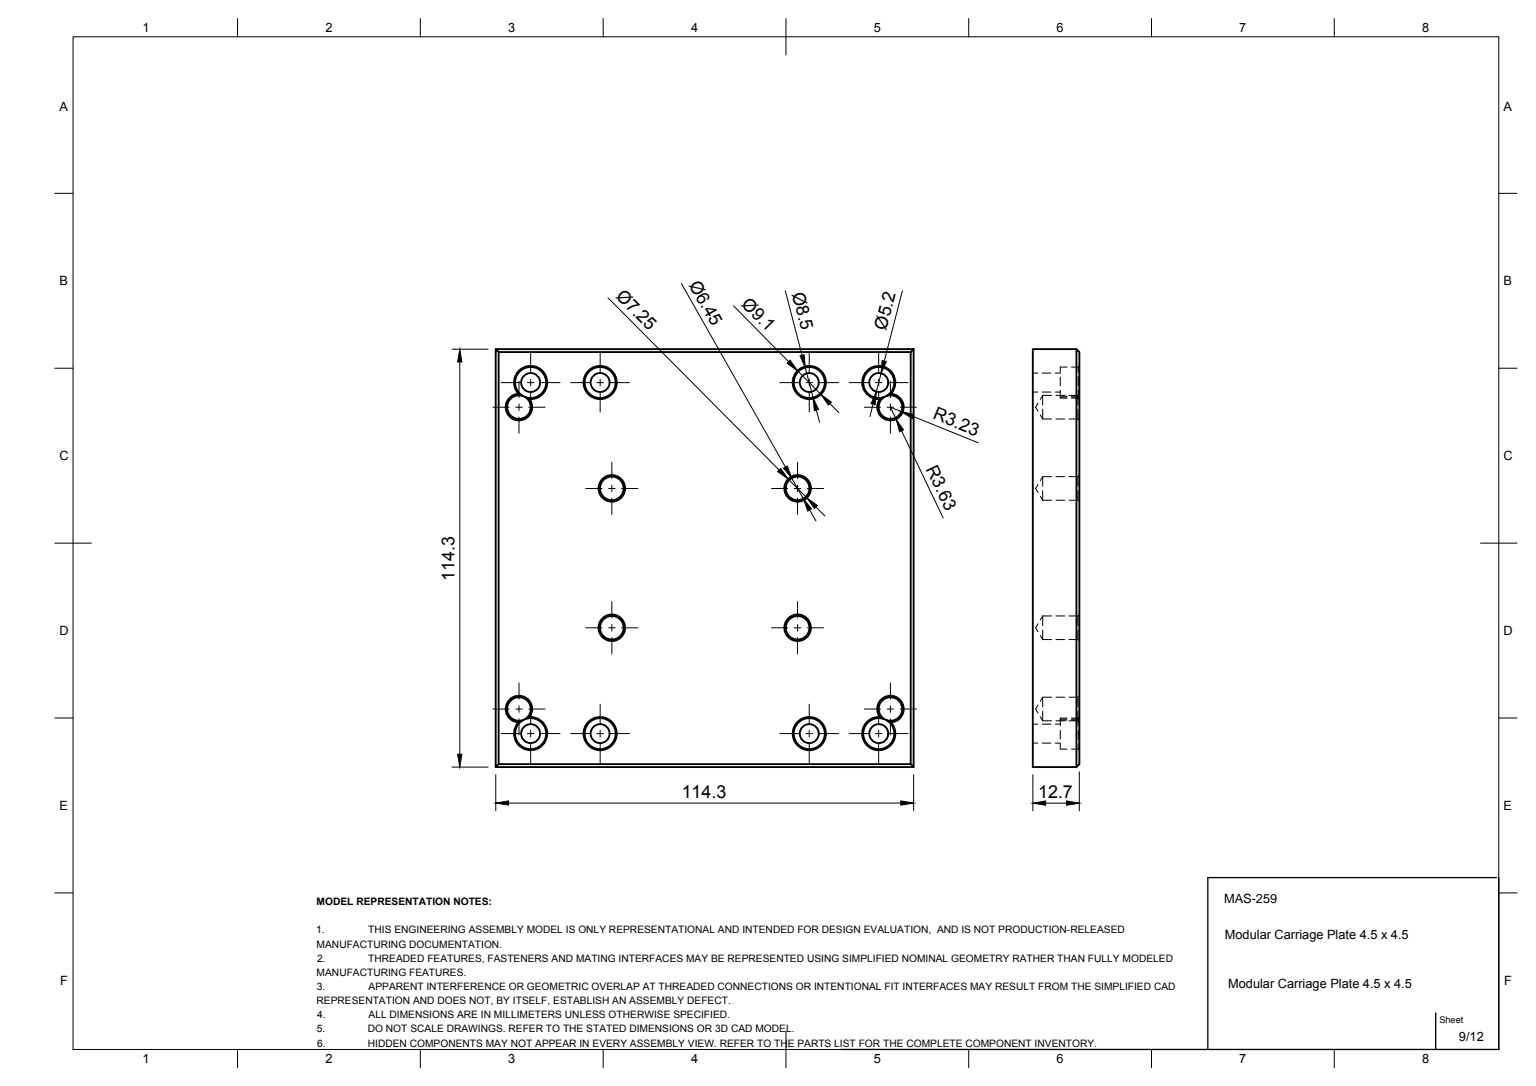
ISO-10303-21;
HEADER;
/* Generated by software containing ST-Developer
 * from STEP Tools, Inc. (www.steptools.com) 
 */

FILE_DESCRIPTION(
/* description */ (''),
/* implementation_level */ '2;1');

FILE_NAME(
/* name */ 'Modular Carriage Plate 4.5 x 4.5.step',
/* time_stamp */ '2026-10-15T13:30:17-07:00',
/* author */ (''),
/* organization */ (''),
/* preprocessor_version */ 'ST-DEVELOPER v20.2',
/* originating_system */ 'Autodesk Translation Framework v15.15.0.0',
/* authorisation */ '');

FILE_SCHEMA (('AUTOMOTIVE_DESIGN { 1 0 10303 214 3 1 1 }'));
ENDSEC;

DATA;
#10=MECHANICAL_DESIGN_GEOMETRIC_PRESENTATION_REPRESENTATION('',(#1034),#71795);
#1014=SHAPE_REPRESENTATION_RELATIONSHIP('SRR','None',#72018,#1024);
#1024=ADVANCED_BREP_SHAPE_REPRESENTATION('',(#1044),#71786);
#1034=STYLED_ITEM('',(#72077),#1044);
#1044=MANIFOLD_SOLID_BREP('Body1',#13636);
#1057=CONICAL_SURFACE('',#13855,4.40000000000001,0.785398163397447);
#1058=CONICAL_SURFACE('',#13874,4.4,0.785398163397434);
#1059=CONICAL_SURFACE('',#13878,4.4,0.78539816339744);
#1060=CONICAL_SURFACE('',#13880,4.4,0.785398163397448);
#1061=CONICAL_SURFACE('',#13884,4.4,0.78539816339744);
#1062=CONICAL_SURFACE('',#13886,4.4,0.785398163397448);
#1063=CONICAL_SURFACE('',#13890,4.4,0.785398163397434);
#1064=CONICAL_SURFACE('',#13894,4.40000000000001,0.785398163397447);
#1065=CONICAL_SURFACE('',#13924,3.42499999999999,0.785398163397437);
#1066=CONICAL_SURFACE('',#13927,3.425,0.785398163397448);
#1067=CONICAL_SURFACE('',#13930,3.425,0.785398163397448);
#1068=CONICAL_SURFACE('',#13933,3.42499999999999,0.785398163397437);
#1069=CONICAL_SURFACE('',#13952,3.42499999999999,0.785398163397437);
#1070=CONICAL_SURFACE('',#13956,3.425,0.785398163397448);
#1071=CONICAL_SURFACE('',#13968,3.425,0.785398163397448);
#1072=CONICAL_SURFACE('',#13972,3.42499999999999,0.785398163397437);
#1073=CONICAL_SURFACE('',#13976,3.225,1.02974425867665);
#1074=CONICAL_SURFACE('',#13977,3.225,1.02974425867665);
#1075=CONICAL_SURFACE('',#13978,3.225,1.02974425867665);
#1076=CONICAL_SURFACE('',#13979,3.225,1.02974425867665);
#1077=CONICAL_SURFACE('',#13980,3.22499999999998,1.02974425867665);
#1078=CONICAL_SURFACE('',#13981,3.22499999999998,1.02974425867665);
#1079=CONICAL_SURFACE('',#13982,3.225,1.02974425867665);
#1080=CONICAL_SURFACE('',#13983,3.225,1.02974425867665);
#1115=B_SPLINE_CURVE_WITH_KNOTS('',3,(#19006,#19007,#19008,#19009,#19010,
#19011),.UNSPECIFIED.,.F.,.F.,(4,2,4),(2.00778188532846,2.05631559190232,
2.12443391712942),.UNSPECIFIED.);
#1116=B_SPLINE_CURVE_WITH_KNOTS('',3,(#19015,#19016,#19017,#19018,#19019,
#19020),.UNSPECIFIED.,.F.,.F.,(4,2,4),(1.74660138399546,1.81470102727558,
1.86325481657749),.UNSPECIFIED.);
#1117=B_SPLINE_CURVE_WITH_KNOTS('',3,(#19070,#19071,#19072,#19073,#19074,
#19075),.UNSPECIFIED.,.F.,.F.,(4,2,4),(2.00778188532849,2.05631559190233,
2.1244339171294),.UNSPECIFIED.);
#1118=B_SPLINE_CURVE_WITH_KNOTS('',3,(#19077,#19078,#19079,#19080,#19081,
#19082),.UNSPECIFIED.,.F.,.F.,(4,2,4),(1.74660138399545,1.81470102727557,
1.86325481657748),.UNSPECIFIED.);
#1119=B_SPLINE_CURVE_WITH_KNOTS('',3,(#19094,#19095,#19096,#19097,#19098,
#19099),.UNSPECIFIED.,.F.,.F.,(4,2,4),(2.00778188532849,2.05631559190233,
2.12443391712941),.UNSPECIFIED.);
#1120=B_SPLINE_CURVE_WITH_KNOTS('',3,(#19101,#19102,#19103,#19104,#19105,
#19106),.UNSPECIFIED.,.F.,.F.,(4,2,4),(1.74660138399546,1.81470102727557,
1.86325481657748),.UNSPECIFIED.);
#1121=B_SPLINE_CURVE_WITH_KNOTS('',3,(#19126,#19127,#19128,#19129,#19130,
#19131),.UNSPECIFIED.,.F.,.F.,(4,2,4),(2.00778188532849,2.05631559190232,
2.1244339171294),.UNSPECIFIED.);
#1122=B_SPLINE_CURVE_WITH_KNOTS('',3,(#19133,#19134,#19135,#19136,#19137,
#19138),.UNSPECIFIED.,.F.,.F.,(4,2,4),(1.74660138399543,1.81470102727559,
1.86325481657752),.UNSPECIFIED.);
#1123=B_SPLINE_CURVE_WITH_KNOTS('',3,(#19142,#19143,#19144,#19145),
 .UNSPECIFIED.,.F.,.F.,(4,4),(-0.456883774528942,-0.419587727931792),
 .UNSPECIFIED.);
#1124=B_SPLINE_CURVE_WITH_KNOTS('',3,(#19152,#19153,#19154,#19155),
 .UNSPECIFIED.,.F.,.F.,(4,4),(-0.557381628443529,-0.520085581846348),
 .UNSPECIFIED.);
#1125=B_SPLINE_CURVE_WITH_KNOTS('',3,(#19168,#19169,#19170,#19171),
 .UNSPECIFIED.,.F.,.F.,(4,4),(-0.456883774528974,-0.419587727931764),
 .UNSPECIFIED.);
#1126=B_SPLINE_CURVE_WITH_KNOTS('',3,(#19178,#19179,#19180,#19181),
 .UNSPECIFIED.,.F.,.F.,(4,4),(-0.557381628443525,-0.520085581846325),
 .UNSPECIFIED.);
#1127=B_SPLINE_CURVE_WITH_KNOTS('',3,(#19191,#19192,#19193,#19194),
 .UNSPECIFIED.,.F.,.F.,(4,4),(-0.456883774528968,-0.419587727931769),
 .UNSPECIFIED.);
#1128=B_SPLINE_CURVE_WITH_KNOTS('',3,(#19201,#19202,#19203,#19204),
 .UNSPECIFIED.,.F.,.F.,(4,4),(-0.557381628443528,-0.52008558184632),
 .UNSPECIFIED.);
#1129=B_SPLINE_CURVE_WITH_KNOTS('',3,(#19214,#19215,#19216,#19217),
 .UNSPECIFIED.,.F.,.F.,(4,4),(-0.456883774528947,-0.419587727931763),
 .UNSPECIFIED.);
#1130=B_SPLINE_CURVE_WITH_KNOTS('',3,(#19224,#19225,#19226,#19227),
 .UNSPECIFIED.,.F.,.F.,(4,4),(-0.557381628443516,-0.520085581846359),
 .UNSPECIFIED.);
#1514=FACE_BOUND('',#2761,.T.);
#1515=FACE_BOUND('',#2762,.T.);
#1516=FACE_BOUND('',#2763,.T.);
#1517=FACE_BOUND('',#2764,.T.);
#1518=FACE_BOUND('',#2765,.T.);
#1519=FACE_BOUND('',#2766,.T.);
#1520=FACE_BOUND('',#2767,.T.);
#1521=FACE_BOUND('',#2768,.T.);
#1522=FACE_BOUND('',#2769,.T.);
#1523=FACE_BOUND('',#2770,.T.);
#1524=FACE_BOUND('',#2771,.T.);
#1525=FACE_BOUND('',#2772,.T.);
#1526=FACE_BOUND('',#2786,.T.);
#1527=FACE_BOUND('',#2788,.T.);
#1528=FACE_BOUND('',#2790,.T.);
#1529=FACE_BOUND('',#2793,.T.);
#1530=FACE_BOUND('',#2795,.T.);
#1531=FACE_BOUND('',#2798,.T.);
#1532=FACE_BOUND('',#2800,.T.);
#1533=FACE_BOUND('',#2803,.T.);
#1534=FACE_BOUND('',#2845,.T.);
#1535=FACE_BOUND('',#2846,.T.);
#1536=FACE_BOUND('',#2847,.T.);
#1537=FACE_BOUND('',#2848,.T.);
#1538=FACE_BOUND('',#2849,.T.);
#1539=FACE_BOUND('',#2850,.T.);
#1540=FACE_BOUND('',#2851,.T.);
#1541=FACE_BOUND('',#2852,.T.);
#1593=PLANE('',#13858);
#1594=PLANE('',#13898);
#1595=PLANE('',#13901);
#1596=PLANE('',#13903);
#1597=PLANE('',#13907);
#1598=PLANE('',#13910);
#1599=PLANE('',#13914);
#1600=PLANE('',#13917);
#1601=PLANE('',#13921);
#1602=PLANE('',#13984);
#1603=PLANE('',#13985);
#1604=PLANE('',#13986);
#1605=PLANE('',#13987);
#1606=PLANE('',#13988);
#1607=PLANE('',#13989);
#1608=PLANE('',#13990);
#1609=PLANE('',#13991);
#1610=PLANE('',#13992);
#2081=FACE_OUTER_BOUND('',#2759,.T.);
#2082=FACE_OUTER_BOUND('',#2760,.T.);
#2083=FACE_OUTER_BOUND('',#2773,.T.);
#2084=FACE_OUTER_BOUND('',#2774,.T.);
#2085=FACE_OUTER_BOUND('',#2775,.T.);
#2086=FACE_OUTER_BOUND('',#2776,.T.);
#2087=FACE_OUTER_BOUND('',#2777,.T.);
#2088=FACE_OUTER_BOUND('',#2778,.T.);
#2089=FACE_OUTER_BOUND('',#2779,.T.);
#2090=FACE_OUTER_BOUND('',#2780,.T.);
#2091=FACE_OUTER_BOUND('',#2781,.T.);
#2092=FACE_OUTER_BOUND('',#2782,.T.);
#2093=FACE_OUTER_BOUND('',#2783,.T.);
#2094=FACE_OUTER_BOUND('',#2784,.T.);
#2095=FACE_OUTER_BOUND('',#2785,.T.);
#2096=FACE_OUTER_BOUND('',#2787,.T.);
#2097=FACE_OUTER_BOUND('',#2789,.T.);
#2098=FACE_OUTER_BOUND('',#2791,.T.);
#2099=FACE_OUTER_BOUND('',#2792,.T.);
#2100=FACE_OUTER_BOUND('',#2794,.T.);
#2101=FACE_OUTER_BOUND('',#2796,.T.);
#2102=FACE_OUTER_BOUND('',#2797,.T.);
#2103=FACE_OUTER_BOUND('',#2799,.T.);
#2104=FACE_OUTER_BOUND('',#2801,.T.);
#2105=FACE_OUTER_BOUND('',#2802,.T.);
#2106=FACE_OUTER_BOUND('',#2804,.T.);
#2107=FACE_OUTER_BOUND('',#2805,.T.);
#2108=FACE_OUTER_BOUND('',#2806,.T.);
#2109=FACE_OUTER_BOUND('',#2807,.T.);
#2110=FACE_OUTER_BOUND('',#2808,.T.);
#2111=FACE_OUTER_BOUND('',#2809,.T.);
#2112=FACE_OUTER_BOUND('',#2810,.T.);
#2113=FACE_OUTER_BOUND('',#2811,.T.);
#2114=FACE_OUTER_BOUND('',#2812,.T.);
#2115=FACE_OUTER_BOUND('',#2813,.T.);
#2116=FACE_OUTER_BOUND('',#2814,.T.);
#2117=FACE_OUTER_BOUND('',#2815,.T.);
#2118=FACE_OUTER_BOUND('',#2816,.T.);
#2119=FACE_OUTER_BOUND('',#2817,.T.);
#2120=FACE_OUTER_BOUND('',#2818,.T.);
#2121=FACE_OUTER_BOUND('',#2819,.T.);
#2122=FACE_OUTER_BOUND('',#2820,.T.);
#2123=FACE_OUTER_BOUND('',#2821,.T.);
#2124=FACE_OUTER_BOUND('',#2822,.T.);
#2125=FACE_OUTER_BOUND('',#2823,.T.);
#2126=FACE_OUTER_BOUND('',#2824,.T.);
#2127=FACE_OUTER_BOUND('',#2825,.T.);
#2128=FACE_OUTER_BOUND('',#2826,.T.);
#2129=FACE_OUTER_BOUND('',#2827,.T.);
#2130=FACE_OUTER_BOUND('',#2828,.T.);
#2131=FACE_OUTER_BOUND('',#2829,.T.);
#2132=FACE_OUTER_BOUND('',#2830,.T.);
#2133=FACE_OUTER_BOUND('',#2831,.T.);
#2134=FACE_OUTER_BOUND('',#2832,.T.);
#2135=FACE_OUTER_BOUND('',#2833,.T.);
#2136=FACE_OUTER_BOUND('',#2834,.T.);
#2137=FACE_OUTER_BOUND('',#2835,.T.);
#2138=FACE_OUTER_BOUND('',#2836,.T.);
#2139=FACE_OUTER_BOUND('',#2837,.T.);
#2140=FACE_OUTER_BOUND('',#2838,.T.);
#2141=FACE_OUTER_BOUND('',#2839,.T.);
#2142=FACE_OUTER_BOUND('',#2840,.T.);
#2143=FACE_OUTER_BOUND('',#2841,.T.);
#2144=FACE_OUTER_BOUND('',#2842,.T.);
#2145=FACE_OUTER_BOUND('',#2843,.T.);
#2146=FACE_OUTER_BOUND('',#2844,.T.);
#2759=EDGE_LOOP('',(#9221,#9222,#9223,#9224));
#2760=EDGE_LOOP('',(#9225,#9226,#9227,#9228));
#2761=EDGE_LOOP('',(#9229));
#2762=EDGE_LOOP('',(#9230));
#2763=EDGE_LOOP('',(#9231));
#2764=EDGE_LOOP('',(#9232));
#2765=EDGE_LOOP('',(#9233,#9234));
#2766=EDGE_LOOP('',(#9235,#9236));
#2767=EDGE_LOOP('',(#9237));
#2768=EDGE_LOOP('',(#9238));
#2769=EDGE_LOOP('',(#9239,#9240));
#2770=EDGE_LOOP('',(#9241,#9242));
#2771=EDGE_LOOP('',(#9243));
#2772=EDGE_LOOP('',(#9244));
#2773=EDGE_LOOP('',(#9245,#9246,#9247,#9248));
#2774=EDGE_LOOP('',(#9249,#9250,#9251,#9252));
#2775=EDGE_LOOP('',(#9253,#9254,#9255,#9256));
#2776=EDGE_LOOP('',(#9257,#9258,#9259,#9260));
#2777=EDGE_LOOP('',(#9261,#9262,#9263,#9264));
#2778=EDGE_LOOP('',(#9265,#9266,#9267,#9268));
#2779=EDGE_LOOP('',(#9269,#9270,#9271,#9272));
#2780=EDGE_LOOP('',(#9273,#9274,#9275,#9276));
#2781=EDGE_LOOP('',(#9277,#9278,#9279,#9280));
#2782=EDGE_LOOP('',(#9281,#9282,#9283,#9284));
#2783=EDGE_LOOP('',(#9285,#9286,#9287,#9288));
#2784=EDGE_LOOP('',(#9289,#9290,#9291,#9292,#9293,#9294));
#2785=EDGE_LOOP('',(#9295,#9296));
#2786=EDGE_LOOP('',(#9297));
#2787=EDGE_LOOP('',(#9298));
#2788=EDGE_LOOP('',(#9299));
#2789=EDGE_LOOP('',(#9300));
#2790=EDGE_LOOP('',(#9301));
#2791=EDGE_LOOP('',(#9302,#9303,#9304,#9305,#9306,#9307));
#2792=EDGE_LOOP('',(#9308,#9309));
#2793=EDGE_LOOP('',(#9310));
#2794=EDGE_LOOP('',(#9311));
#2795=EDGE_LOOP('',(#9312));
#2796=EDGE_LOOP('',(#9313,#9314,#9315,#9316,#9317,#9318));
#2797=EDGE_LOOP('',(#9319,#9320));
#2798=EDGE_LOOP('',(#9321));
#2799=EDGE_LOOP('',(#9322));
#2800=EDGE_LOOP('',(#9323));
#2801=EDGE_LOOP('',(#9324,#9325,#9326,#9327,#9328,#9329));
#2802=EDGE_LOOP('',(#9330,#9331));
#2803=EDGE_LOOP('',(#9332));
#2804=EDGE_LOOP('',(#9333,#9334,#9335,#9336,#9337,#9338,#9339));
#2805=EDGE_LOOP('',(#9340,#9341,#9342,#9343,#9344,#9345,#9346));
#2806=EDGE_LOOP('',(#9347,#9348,#9349,#9350,#9351,#9352,#9353));
#2807=EDGE_LOOP('',(#9354,#9355,#9356,#9357,#9358,#9359,#9360));
#2808=EDGE_LOOP('',(#9361,#9362,#9363,#9364));
#2809=EDGE_LOOP('',(#9365,#9366,#9367,#9368));
#2810=EDGE_LOOP('',(#9369,#9370,#9371,#9372));
#2811=EDGE_LOOP('',(#9373,#9374,#9375,#9376));
#2812=EDGE_LOOP('',(#9377,#9378,#9379,#9380));
#2813=EDGE_LOOP('',(#9381,#9382,#9383,#9384));
#2814=EDGE_LOOP('',(#9385,#9386,#9387,#9388));
#2815=EDGE_LOOP('',(#9389,#9390,#9391,#9392));
#2816=EDGE_LOOP('',(#9393,#9394,#9395,#9396));
#2817=EDGE_LOOP('',(#9397,#9398,#9399,#9400));
#2818=EDGE_LOOP('',(#9401,#9402,#9403,#9404));
#2819=EDGE_LOOP('',(#9405,#9406,#9407,#9408));
#2820=EDGE_LOOP('',(#9409,#9410,#9411,#9412,#9413,#9414,#9415,#9416));
#2821=EDGE_LOOP('',(#9417,#9418,#9419,#9420,#9421,#9422,#9423,#9424));
#2822=EDGE_LOOP('',(#9425,#9426,#9427,#9428,#9429,#9430,#9431,#9432));
#2823=EDGE_LOOP('',(#9433,#9434,#9435,#9436,#9437,#9438,#9439,#9440));
#2824=EDGE_LOOP('',(#9441,#9442,#9443,#9444));
#2825=EDGE_LOOP('',(#9445,#9446,#9447,#9448));
#2826=EDGE_LOOP('',(#9449,#9450,#9451,#9452));
#2827=EDGE_LOOP('',(#9453,#9454,#9455,#9456));
#2828=EDGE_LOOP('',(#9457,#9458,#9459));
#2829=EDGE_LOOP('',(#9460,#9461,#9462));
#2830=EDGE_LOOP('',(#9463,#9464,#9465));
#2831=EDGE_LOOP('',(#9466,#9467,#9468));
#2832=EDGE_LOOP('',(#9469,#9470,#9471));
#2833=EDGE_LOOP('',(#9472,#9473,#9474));
#2834=EDGE_LOOP('',(#9475,#9476,#9477));
#2835=EDGE_LOOP('',(#9478,#9479,#9480));
#2836=EDGE_LOOP('',(#9481,#9482,#9483,#9484));
#2837=EDGE_LOOP('',(#9485,#9486,#9487,#9488));
#2838=EDGE_LOOP('',(#9489,#9490,#9491,#9492));
#2839=EDGE_LOOP('',(#9493,#9494,#9495,#9496));
#2840=EDGE_LOOP('',(#9497,#9498,#9499,#9500));
#2841=EDGE_LOOP('',(#9501,#9502,#9503,#9504));
#2842=EDGE_LOOP('',(#9505,#9506,#9507,#9508));
#2843=EDGE_LOOP('',(#9509,#9510,#9511,#9512));
#2844=EDGE_LOOP('',(#9513,#9514,#9515,#9516));
#2845=EDGE_LOOP('',(#9517));
#2846=EDGE_LOOP('',(#9518));
#2847=EDGE_LOOP('',(#9519));
#2848=EDGE_LOOP('',(#9520));
#2849=EDGE_LOOP('',(#9521));
#2850=EDGE_LOOP('',(#9522));
#2851=EDGE_LOOP('',(#9523));
#2852=EDGE_LOOP('',(#9524));
#3440=CIRCLE('',#13856,4.55000000000001);
#3441=CIRCLE('',#13857,4.25000000000001);
#3442=CIRCLE('',#13859,4.55);
#3443=CIRCLE('',#13860,4.55);
#3444=CIRCLE('',#13861,4.55);
#3445=CIRCLE('',#13862,3.625);
#3446=CIRCLE('',#13863,4.55000000000001);
#3447=CIRCLE('',#13864,3.62499999999999);
#3448=CIRCLE('',#13865,3.62499999999999);
#3449=CIRCLE('',#13866,3.62499999999999);
#3450=CIRCLE('',#13867,3.625);
#3451=CIRCLE('',#13868,4.55);
#3452=CIRCLE('',#13869,3.625);
#3453=CIRCLE('',#13870,4.55);
#3454=CIRCLE('',#13871,3.625);
#3455=CIRCLE('',#13872,3.62499999999999);
#3456=CIRCLE('',#13873,4.55);
#3457=CIRCLE('',#13875,4.25000000000001);
#3458=CIRCLE('',#13877,4.25000000000001);
#3459=CIRCLE('',#13879,4.25);
#3460=CIRCLE('',#13881,4.25);
#3461=CIRCLE('',#13883,4.25);
#3462=CIRCLE('',#13885,4.25);
#3463=CIRCLE('',#13887,4.25);
#3464=CIRCLE('',#13889,4.25);
#3465=CIRCLE('',#13891,4.25000000000001);
#3466=CIRCLE('',#13893,4.25000000000001);
#3467=CIRCLE('',#13895,4.25000000000001);
#3468=CIRCLE('',#13897,4.25000000000001);
#3469=CIRCLE('',#13899,3.225);
#3470=CIRCLE('',#13900,2.6);
#3471=CIRCLE('',#13902,2.6);
#3472=CIRCLE('',#13904,2.6);
#3473=CIRCLE('',#13906,4.25);
#3474=CIRCLE('',#13908,3.225);
#3475=CIRCLE('',#13909,2.6);
#3476=CIRCLE('',#13911,2.6);
#3477=CIRCLE('',#13913,4.25);
#3478=CIRCLE('',#13915,3.225);
#3479=CIRCLE('',#13916,2.6);
#3480=CIRCLE('',#13918,2.6);
#3481=CIRCLE('',#13920,4.25000000000001);
#3482=CIRCLE('',#13922,3.225);
#3483=CIRCLE('',#13923,2.6);
#3484=CIRCLE('',#13925,3.225);
#3485=CIRCLE('',#13926,3.225);
#3486=CIRCLE('',#13928,3.225);
#3487=CIRCLE('',#13929,3.225);
#3488=CIRCLE('',#13931,3.225);
#3489=CIRCLE('',#13932,3.225);
#3490=CIRCLE('',#13934,3.225);
#3491=CIRCLE('',#13935,3.225);
#3492=CIRCLE('',#13937,2.6);
#3493=CIRCLE('',#13939,2.6);
#3494=CIRCLE('',#13941,2.6);
#3495=CIRCLE('',#13943,2.6);
#3496=CIRCLE('',#13945,2.6);
#3497=CIRCLE('',#13947,2.6);
#3498=CIRCLE('',#13949,2.6);
#3499=CIRCLE('',#13951,2.6);
#3500=CIRCLE('',#13953,3.225);
#3501=CIRCLE('',#13955,3.225);
#3502=CIRCLE('',#13957,3.225);
#3503=CIRCLE('',#13959,3.225);
#3504=CIRCLE('',#13961,3.225);
#3505=CIRCLE('',#13963,3.225);
#3506=CIRCLE('',#13965,3.225);
#3507=CIRCLE('',#13967,3.225);
#3508=CIRCLE('',#13969,3.225);
#3509=CIRCLE('',#13971,3.225);
#3510=CIRCLE('',#13973,3.225);
#3511=CIRCLE('',#13975,3.225);
#3912=LINE('',#19025,#4823);
#3913=LINE('',#19027,#4824);
#3914=LINE('',#19029,#4825);
#3915=LINE('',#19030,#4826);
#3916=LINE('',#19063,#4827);
#3917=LINE('',#19066,#4828);
#3918=LINE('',#19087,#4829);
#3919=LINE('',#19090,#4830);
#3920=LINE('',#19111,#4831);
#3921=LINE('',#19114,#4832);
#3922=LINE('',#19119,#4833);
#3923=LINE('',#19122,#4834);
#3924=LINE('',#19147,#4835);
#3925=LINE('',#19151,#4836);
#3926=LINE('',#19173,#4837);
#3927=LINE('',#19177,#4838);
#3928=LINE('',#19196,#4839);
#3929=LINE('',#19200,#4840);
#3930=LINE('',#19219,#4841);
#3931=LINE('',#19223,#4842);
#3932=LINE('',#19250,#4843);
#3933=LINE('',#19254,#4844);
#3934=LINE('',#19258,#4845);
#3935=LINE('',#19262,#4846);
#3936=LINE('',#19266,#4847);
#3937=LINE('',#19270,#4848);
#3938=LINE('',#19274,#4849);
#3939=LINE('',#19278,#4850);
#3940=LINE('',#19283,#4851);
#3941=LINE('',#19286,#4852);
#3942=LINE('',#19291,#4853);
#3943=LINE('',#19294,#4854);
#3944=LINE('',#19298,#4855);
#3945=LINE('',#19302,#4856);
#3946=LINE('',#19306,#4857);
#3947=LINE('',#19310,#4858);
#3948=LINE('',#19315,#4859);
#3949=LINE('',#19318,#4860);
#3950=LINE('',#19323,#4861);
#3951=LINE('',#19326,#4862);
#3952=LINE('',#19330,#4863);
#3953=LINE('',#19333,#4864);
#3954=LINE('',#19336,#4865);
#3955=LINE('',#19339,#4866);
#3956=LINE('',#19342,#4867);
#3957=LINE('',#19345,#4868);
#3958=LINE('',#19348,#4869);
#3959=LINE('',#19351,#4870);
#3960=LINE('',#19354,#4871);
#3961=LINE('',#19356,#4872);
#3962=LINE('',#19357,#4873);
#3963=LINE('',#19360,#4874);
#3964=LINE('',#19361,#4875);
#3965=LINE('',#19364,#4876);
#3966=LINE('',#19365,#4877);
#3967=LINE('',#19367,#4878);
#3968=LINE('',#19370,#4879);
#3969=LINE('',#19372,#4880);
#3970=LINE('',#19373,#4881);
#3971=LINE('',#19376,#4882);
#3972=LINE('',#19377,#4883);
#3973=LINE('',#19380,#4884);
#3974=LINE('',#19381,#4885);
#3975=LINE('',#19383,#4886);
#4823=VECTOR('',#15323,10.);
#4824=VECTOR('',#15324,10.);
#4825=VECTOR('',#15325,10.);
#4826=VECTOR('',#15326,10.);
#4827=VECTOR('',#15361,4.4);
#4828=VECTOR('',#15364,4.25000000000001);
#4829=VECTOR('',#15375,4.4);
#4830=VECTOR('',#15378,4.25);
#4831=VECTOR('',#15389,4.4);
#4832=VECTOR('',#15392,4.25);
#4833=VECTOR('',#15399,4.4);
#4834=VECTOR('',#15402,4.25000000000001);
#4835=VECTOR('',#15411,10.);
#4836=VECTOR('',#15414,10.);
#4837=VECTOR('',#15431,10.);
#4838=VECTOR('',#15434,10.);
#4839=VECTOR('',#15447,10.);
#4840=VECTOR('',#15450,10.);
#4841=VECTOR('',#15463,10.);
#4842=VECTOR('',#15466,10.);
#4843=VECTOR('',#15499,2.6);
#4844=VECTOR('',#15504,2.6);
#4845=VECTOR('',#15509,2.6);
#4846=VECTOR('',#15514,2.6);
#4847=VECTOR('',#15519,2.6);
#4848=VECTOR('',#15524,2.6);
#4849=VECTOR('',#15529,2.6);
#4850=VECTOR('',#15534,2.6);
#4851=VECTOR('',#15541,3.42499999999999);
#4852=VECTOR('',#15544,3.225);
#4853=VECTOR('',#15551,3.425);
#4854=VECTOR('',#15554,3.225);
#4855=VECTOR('',#15559,3.225);
#4856=VECTOR('',#15564,3.225);
#4857=VECTOR('',#15569,3.225);
#4858=VECTOR('',#15574,3.225);
#4859=VECTOR('',#15581,3.425);
#4860=VECTOR('',#15584,3.225);
#4861=VECTOR('',#15591,3.42499999999999);
#4862=VECTOR('',#15594,3.225);
#4863=VECTOR('',#15599,3.225);
#4864=VECTOR('',#15602,3.225);
#4865=VECTOR('',#15605,3.225);
#4866=VECTOR('',#15608,3.225);
#4867=VECTOR('',#15611,3.22499999999998);
#4868=VECTOR('',#15614,3.22499999999998);
#4869=VECTOR('',#15617,3.225);
#4870=VECTOR('',#15620,3.225);
#4871=VECTOR('',#15623,10.);
#4872=VECTOR('',#15624,10.);
#4873=VECTOR('',#15625,10.);
#4874=VECTOR('',#15628,10.);
#4875=VECTOR('',#15629,10.);
#4876=VECTOR('',#15632,10.);
#4877=VECTOR('',#15633,10.);
#4878=VECTOR('',#15636,10.);
#4879=VECTOR('',#15639,10.);
#4880=VECTOR('',#15640,10.);
#4881=VECTOR('',#15641,10.);
#4882=VECTOR('',#15644,10.);
#4883=VECTOR('',#15645,10.);
#4884=VECTOR('',#15648,10.);
#4885=VECTOR('',#15649,10.);
#4886=VECTOR('',#15652,10.);
#5752=VERTEX_POINT('',#19004);
#5753=VERTEX_POINT('',#19005);
#5754=VERTEX_POINT('',#19012);
#5755=VERTEX_POINT('',#19014);
#5756=VERTEX_POINT('',#19023);
#5757=VERTEX_POINT('',#19024);
#5758=VERTEX_POINT('',#19026);
#5759=VERTEX_POINT('',#19028);
#5760=VERTEX_POINT('',#19031);
#5761=VERTEX_POINT('',#19033);
#5762=VERTEX_POINT('',#19035);
#5763=VERTEX_POINT('',#19037);
#5764=VERTEX_POINT('',#19039);
#5765=VERTEX_POINT('',#19040);
#5766=VERTEX_POINT('',#19044);
#5767=VERTEX_POINT('',#19046);
#5768=VERTEX_POINT('',#19048);
#5769=VERTEX_POINT('',#19049);
#5770=VERTEX_POINT('',#19052);
#5771=VERTEX_POINT('',#19053);
#5772=VERTEX_POINT('',#19056);
#5773=VERTEX_POINT('',#19058);
#5774=VERTEX_POINT('',#19061);
#5775=VERTEX_POINT('',#19065);
#5776=VERTEX_POINT('',#19069);
#5777=VERTEX_POINT('',#19076);
#5778=VERTEX_POINT('',#19085);
#5779=VERTEX_POINT('',#19089);
#5780=VERTEX_POINT('',#19093);
#5781=VERTEX_POINT('',#19100);
#5782=VERTEX_POINT('',#19109);
#5783=VERTEX_POINT('',#19113);
#5784=VERTEX_POINT('',#19117);
#5785=VERTEX_POINT('',#19121);
#5786=VERTEX_POINT('',#19125);
#5787=VERTEX_POINT('',#19132);
#5788=VERTEX_POINT('',#19141);
#5789=VERTEX_POINT('',#19146);
#5790=VERTEX_POINT('',#19148);
#5791=VERTEX_POINT('',#19150);
#5792=VERTEX_POINT('',#19158);
#5793=VERTEX_POINT('',#19161);
#5794=VERTEX_POINT('',#19164);
#5795=VERTEX_POINT('',#19167);
#5796=VERTEX_POINT('',#19172);
#5797=VERTEX_POINT('',#19174);
#5798=VERTEX_POINT('',#19176);
#5799=VERTEX_POINT('',#19184);
#5800=VERTEX_POINT('',#19187);
#5801=VERTEX_POINT('',#19190);
#5802=VERTEX_POINT('',#19195);
#5803=VERTEX_POINT('',#19197);
#5804=VERTEX_POINT('',#19199);
#5805=VERTEX_POINT('',#19207);
#5806=VERTEX_POINT('',#19210);
#5807=VERTEX_POINT('',#19213);
#5808=VERTEX_POINT('',#19218);
#5809=VERTEX_POINT('',#19220);
#5810=VERTEX_POINT('',#19222);
#5811=VERTEX_POINT('',#19230);
#5812=VERTEX_POINT('',#19233);
#5813=VERTEX_POINT('',#19237);
#5814=VERTEX_POINT('',#19241);
#5815=VERTEX_POINT('',#19245);
#5816=VERTEX_POINT('',#19249);
#5817=VERTEX_POINT('',#19253);
#5818=VERTEX_POINT('',#19257);
#5819=VERTEX_POINT('',#19261);
#5820=VERTEX_POINT('',#19265);
#5821=VERTEX_POINT('',#19269);
#5822=VERTEX_POINT('',#19273);
#5823=VERTEX_POINT('',#19277);
#5824=VERTEX_POINT('',#19281);
#5825=VERTEX_POINT('',#19285);
#5826=VERTEX_POINT('',#19289);
#5827=VERTEX_POINT('',#19293);
#5828=VERTEX_POINT('',#19297);
#5829=VERTEX_POINT('',#19301);
#5830=VERTEX_POINT('',#19305);
#5831=VERTEX_POINT('',#19309);
#5832=VERTEX_POINT('',#19313);
#5833=VERTEX_POINT('',#19317);
#5834=VERTEX_POINT('',#19321);
#5835=VERTEX_POINT('',#19325);
#5836=VERTEX_POINT('',#19329);
#5837=VERTEX_POINT('',#19332);
#5838=VERTEX_POINT('',#19335);
#5839=VERTEX_POINT('',#19338);
#5840=VERTEX_POINT('',#19341);
#5841=VERTEX_POINT('',#19344);
#5842=VERTEX_POINT('',#19347);
#5843=VERTEX_POINT('',#19350);
#5844=VERTEX_POINT('',#19353);
#5845=VERTEX_POINT('',#19355);
#5846=VERTEX_POINT('',#19359);
#5847=VERTEX_POINT('',#19363);
#5848=VERTEX_POINT('',#19369);
#5849=VERTEX_POINT('',#19371);
#5850=VERTEX_POINT('',#19375);
#5851=VERTEX_POINT('',#19379);
#7145=EDGE_CURVE('',#5752,#5753,#1115,.T.);
#7146=EDGE_CURVE('',#5753,#5754,#3440,.T.);
#7147=EDGE_CURVE('',#5754,#5755,#1116,.T.);
#7148=EDGE_CURVE('',#5755,#5752,#3441,.T.);
#7149=EDGE_CURVE('',#5756,#5757,#3912,.T.);
#7150=EDGE_CURVE('',#5758,#5756,#3913,.T.);
#7151=EDGE_CURVE('',#5759,#5758,#3914,.T.);
#7152=EDGE_CURVE('',#5757,#5759,#3915,.T.);
#7153=EDGE_CURVE('',#5760,#5760,#3442,.T.);
#7154=EDGE_CURVE('',#5761,#5761,#3443,.T.);
#7155=EDGE_CURVE('',#5762,#5762,#3444,.T.);
#7156=EDGE_CURVE('',#5763,#5763,#3445,.T.);
#7157=EDGE_CURVE('',#5764,#5765,#3446,.T.);
#7158=EDGE_CURVE('',#5765,#5764,#3447,.T.);
#7159=EDGE_CURVE('',#5754,#5753,#3448,.T.);
#7160=EDGE_CURVE('',#5766,#5766,#3449,.T.);
#7161=EDGE_CURVE('',#5767,#5767,#3450,.T.);
#7162=EDGE_CURVE('',#5768,#5769,#3451,.T.);
#7163=EDGE_CURVE('',#5769,#5768,#3452,.T.);
#7164=EDGE_CURVE('',#5770,#5771,#3453,.T.);
#7165=EDGE_CURVE('',#5771,#5770,#3454,.T.);
#7166=EDGE_CURVE('',#5772,#5772,#3455,.T.);
#7167=EDGE_CURVE('',#5773,#5773,#3456,.T.);
#7168=EDGE_CURVE('',#5774,#5774,#3457,.T.);
#7169=EDGE_CURVE('',#5774,#5760,#3916,.T.);
#7170=EDGE_CURVE('',#5774,#5775,#3917,.T.);
#7171=EDGE_CURVE('',#5775,#5775,#3458,.T.);
#7172=EDGE_CURVE('',#5776,#5770,#1117,.T.);
#7173=EDGE_CURVE('',#5771,#5777,#1118,.T.);
#7174=EDGE_CURVE('',#5777,#5776,#3459,.T.);
#7175=EDGE_CURVE('',#5778,#5778,#3460,.T.);
#7176=EDGE_CURVE('',#5778,#5761,#3918,.T.);
#7177=EDGE_CURVE('',#5778,#5779,#3919,.T.);
#7178=EDGE_CURVE('',#5779,#5779,#3461,.T.);
#7179=EDGE_CURVE('',#5780,#5768,#1119,.T.);
#7180=EDGE_CURVE('',#5769,#5781,#1120,.T.);
#7181=EDGE_CURVE('',#5781,#5780,#3462,.T.);
#7182=EDGE_CURVE('',#5782,#5782,#3463,.T.);
#7183=EDGE_CURVE('',#5782,#5762,#3920,.T.);
#7184=EDGE_CURVE('',#5782,#5783,#3921,.T.);
#7185=EDGE_CURVE('',#5783,#5783,#3464,.T.);
#7186=EDGE_CURVE('',#5784,#5784,#3465,.T.);
#7187=EDGE_CURVE('',#5784,#5773,#3922,.T.);
#7188=EDGE_CURVE('',#5784,#5785,#3923,.T.);
#7189=EDGE_CURVE('',#5785,#5785,#3466,.T.);
#7190=EDGE_CURVE('',#5786,#5764,#1121,.T.);
#7191=EDGE_CURVE('',#5765,#5787,#1122,.T.);
#7192=EDGE_CURVE('',#5787,#5786,#3467,.T.);
#7193=EDGE_CURVE('',#5788,#5787,#1123,.T.);
#7194=EDGE_CURVE('',#5789,#5788,#3924,.T.);
#7195=EDGE_CURVE('',#5789,#5790,#3468,.T.);
#7196=EDGE_CURVE('',#5791,#5790,#3925,.T.);
#7197=EDGE_CURVE('',#5786,#5791,#1124,.T.);
#7198=EDGE_CURVE('',#5790,#5789,#3469,.T.);
#7199=EDGE_CURVE('',#5792,#5792,#3470,.T.);
#7200=EDGE_CURVE('',#5793,#5793,#3471,.T.);
#7201=EDGE_CURVE('',#5794,#5794,#3472,.T.);
#7202=EDGE_CURVE('',#5795,#5781,#1125,.T.);
#7203=EDGE_CURVE('',#5796,#5795,#3926,.T.);
#7204=EDGE_CURVE('',#5796,#5797,#3473,.T.);
#7205=EDGE_CURVE('',#5798,#5797,#3927,.T.);
#7206=EDGE_CURVE('',#5780,#5798,#1126,.T.);
#7207=EDGE_CURVE('',#5797,#5796,#3474,.T.);
#7208=EDGE_CURVE('',#5799,#5799,#3475,.T.);
#7209=EDGE_CURVE('',#5800,#5800,#3476,.T.);
#7210=EDGE_CURVE('',#5801,#5777,#1127,.T.);
#7211=EDGE_CURVE('',#5802,#5801,#3928,.T.);
#7212=EDGE_CURVE('',#5802,#5803,#3477,.T.);
#7213=EDGE_CURVE('',#5804,#5803,#3929,.T.);
#7214=EDGE_CURVE('',#5776,#5804,#1128,.T.);
#7215=EDGE_CURVE('',#5803,#5802,#3478,.T.);
#7216=EDGE_CURVE('',#5805,#5805,#3479,.T.);
#7217=EDGE_CURVE('',#5806,#5806,#3480,.T.);
#7218=EDGE_CURVE('',#5807,#5755,#1129,.T.);
#7219=EDGE_CURVE('',#5808,#5807,#3930,.T.);
#7220=EDGE_CURVE('',#5808,#5809,#3481,.T.);
#7221=EDGE_CURVE('',#5810,#5809,#3931,.T.);
#7222=EDGE_CURVE('',#5752,#5810,#1130,.T.);
#7223=EDGE_CURVE('',#5809,#5808,#3482,.T.);
#7224=EDGE_CURVE('',#5811,#5811,#3483,.T.);
#7225=EDGE_CURVE('',#5791,#5812,#3484,.T.);
#7226=EDGE_CURVE('',#5812,#5788,#3485,.T.);
#7227=EDGE_CURVE('',#5798,#5813,#3486,.T.);
#7228=EDGE_CURVE('',#5813,#5795,#3487,.T.);
#7229=EDGE_CURVE('',#5804,#5814,#3488,.T.);
#7230=EDGE_CURVE('',#5814,#5801,#3489,.T.);
#7231=EDGE_CURVE('',#5810,#5815,#3490,.T.);
#7232=EDGE_CURVE('',#5815,#5807,#3491,.T.);
#7233=EDGE_CURVE('',#5792,#5816,#3932,.T.);
#7234=EDGE_CURVE('',#5816,#5816,#3492,.T.);
#7235=EDGE_CURVE('',#5793,#5817,#3933,.T.);
#7236=EDGE_CURVE('',#5817,#5817,#3493,.T.);
#7237=EDGE_CURVE('',#5794,#5818,#3934,.T.);
#7238=EDGE_CURVE('',#5818,#5818,#3494,.T.);
#7239=EDGE_CURVE('',#5799,#5819,#3935,.T.);
#7240=EDGE_CURVE('',#5819,#5819,#3495,.T.);
#7241=EDGE_CURVE('',#5800,#5820,#3936,.T.);
#7242=EDGE_CURVE('',#5820,#5820,#3496,.T.);
#7243=EDGE_CURVE('',#5805,#5821,#3937,.T.);
#7244=EDGE_CURVE('',#5821,#5821,#3497,.T.);
#7245=EDGE_CURVE('',#5806,#5822,#3938,.T.);
#7246=EDGE_CURVE('',#5822,#5822,#3498,.T.);
#7247=EDGE_CURVE('',#5811,#5823,#3939,.T.);
#7248=EDGE_CURVE('',#5823,#5823,#3499,.T.);
#7249=EDGE_CURVE('',#5824,#5824,#3500,.T.);
#7250=EDGE_CURVE('',#5824,#5772,#3940,.T.);
#7251=EDGE_CURVE('',#5824,#5825,#3941,.T.);
#7252=EDGE_CURVE('',#5825,#5825,#3501,.T.);
#7253=EDGE_CURVE('',#5826,#5826,#3502,.T.);
#7254=EDGE_CURVE('',#5826,#5763,#3942,.T.);
#7255=EDGE_CURVE('',#5826,#5827,#3943,.T.);
#7256=EDGE_CURVE('',#5827,#5827,#3503,.T.);
#7257=EDGE_CURVE('',#5814,#5828,#3944,.T.);
#7258=EDGE_CURVE('',#5828,#5828,#3504,.T.);
#7259=EDGE_CURVE('',#5812,#5829,#3945,.T.);
#7260=EDGE_CURVE('',#5829,#5829,#3505,.T.);
#7261=EDGE_CURVE('',#5813,#5830,#3946,.T.);
#7262=EDGE_CURVE('',#5830,#5830,#3506,.T.);
#7263=EDGE_CURVE('',#5815,#5831,#3947,.T.);
#7264=EDGE_CURVE('',#5831,#5831,#3507,.T.);
#7265=EDGE_CURVE('',#5832,#5832,#3508,.T.);
#7266=EDGE_CURVE('',#5832,#5767,#3948,.T.);
#7267=EDGE_CURVE('',#5832,#5833,#3949,.T.);
#7268=EDGE_CURVE('',#5833,#5833,#3509,.T.);
#7269=EDGE_CURVE('',#5834,#5834,#3510,.T.);
#7270=EDGE_CURVE('',#5834,#5766,#3950,.T.);
#7271=EDGE_CURVE('',#5834,#5835,#3951,.T.);
#7272=EDGE_CURVE('',#5835,#5835,#3511,.T.);
#7273=EDGE_CURVE('',#5836,#5825,#3952,.T.);
#7274=EDGE_CURVE('',#5837,#5835,#3953,.T.);
#7275=EDGE_CURVE('',#5838,#5827,#3954,.T.);
#7276=EDGE_CURVE('',#5839,#5833,#3955,.T.);
#7277=EDGE_CURVE('',#5840,#5831,#3956,.T.);
#7278=EDGE_CURVE('',#5841,#5829,#3957,.T.);
#7279=EDGE_CURVE('',#5842,#5830,#3958,.T.);
#7280=EDGE_CURVE('',#5843,#5828,#3959,.T.);
#7281=EDGE_CURVE('',#5757,#5844,#3960,.T.);
#7282=EDGE_CURVE('',#5844,#5845,#3961,.T.);
#7283=EDGE_CURVE('',#5756,#5845,#3962,.T.);
#7284=EDGE_CURVE('',#5759,#5846,#3963,.T.);
#7285=EDGE_CURVE('',#5846,#5844,#3964,.T.);
#7286=EDGE_CURVE('',#5758,#5847,#3965,.T.);
#7287=EDGE_CURVE('',#5847,#5846,#3966,.T.);
#7288=EDGE_CURVE('',#5845,#5847,#3967,.T.);
#7289=EDGE_CURVE('',#5848,#5845,#3968,.T.);
#7290=EDGE_CURVE('',#5849,#5848,#3969,.T.);
#7291=EDGE_CURVE('',#5849,#5847,#3970,.T.);
#7292=EDGE_CURVE('',#5850,#5844,#3971,.T.);
#7293=EDGE_CURVE('',#5848,#5850,#3972,.T.);
#7294=EDGE_CURVE('',#5851,#5849,#3973,.T.);
#7295=EDGE_CURVE('',#5851,#5846,#3974,.T.);
#7296=EDGE_CURVE('',#5850,#5851,#3975,.T.);
#9221=ORIENTED_EDGE('',*,*,#7145,.T.);
#9222=ORIENTED_EDGE('',*,*,#7146,.T.);
#9223=ORIENTED_EDGE('',*,*,#7147,.T.);
#9224=ORIENTED_EDGE('',*,*,#7148,.T.);
#9225=ORIENTED_EDGE('',*,*,#7149,.F.);
#9226=ORIENTED_EDGE('',*,*,#7150,.F.);
#9227=ORIENTED_EDGE('',*,*,#7151,.F.);
#9228=ORIENTED_EDGE('',*,*,#7152,.F.);
#9229=ORIENTED_EDGE('',*,*,#7153,.F.);
#9230=ORIENTED_EDGE('',*,*,#7154,.F.);
#9231=ORIENTED_EDGE('',*,*,#7155,.F.);
#9232=ORIENTED_EDGE('',*,*,#7156,.F.);
#9233=ORIENTED_EDGE('',*,*,#7157,.F.);
#9234=ORIENTED_EDGE('',*,*,#7158,.F.);
#9235=ORIENTED_EDGE('',*,*,#7146,.F.);
#9236=ORIENTED_EDGE('',*,*,#7159,.F.);
#9237=ORIENTED_EDGE('',*,*,#7160,.F.);
#9238=ORIENTED_EDGE('',*,*,#7161,.F.);
#9239=ORIENTED_EDGE('',*,*,#7162,.F.);
#9240=ORIENTED_EDGE('',*,*,#7163,.F.);
#9241=ORIENTED_EDGE('',*,*,#7164,.F.);
#9242=ORIENTED_EDGE('',*,*,#7165,.F.);
#9243=ORIENTED_EDGE('',*,*,#7166,.F.);
#9244=ORIENTED_EDGE('',*,*,#7167,.F.);
#9245=ORIENTED_EDGE('',*,*,#7168,.T.);
#9246=ORIENTED_EDGE('',*,*,#7169,.T.);
#9247=ORIENTED_EDGE('',*,*,#7153,.T.);
#9248=ORIENTED_EDGE('',*,*,#7169,.F.);
#9249=ORIENTED_EDGE('',*,*,#7168,.F.);
#9250=ORIENTED_EDGE('',*,*,#7170,.T.);
#9251=ORIENTED_EDGE('',*,*,#7171,.T.);
#9252=ORIENTED_EDGE('',*,*,#7170,.F.);
#9253=ORIENTED_EDGE('',*,*,#7172,.T.);
#9254=ORIENTED_EDGE('',*,*,#7164,.T.);
#9255=ORIENTED_EDGE('',*,*,#7173,.T.);
#9256=ORIENTED_EDGE('',*,*,#7174,.T.);
#9257=ORIENTED_EDGE('',*,*,#7175,.T.);
#9258=ORIENTED_EDGE('',*,*,#7176,.T.);
#9259=ORIENTED_EDGE('',*,*,#7154,.T.);
#9260=ORIENTED_EDGE('',*,*,#7176,.F.);
#9261=ORIENTED_EDGE('',*,*,#7175,.F.);
#9262=ORIENTED_EDGE('',*,*,#7177,.T.);
#9263=ORIENTED_EDGE('',*,*,#7178,.T.);
#9264=ORIENTED_EDGE('',*,*,#7177,.F.);
#9265=ORIENTED_EDGE('',*,*,#7179,.T.);
#9266=ORIENTED_EDGE('',*,*,#7162,.T.);
#9267=ORIENTED_EDGE('',*,*,#7180,.T.);
#9268=ORIENTED_EDGE('',*,*,#7181,.T.);
#9269=ORIENTED_EDGE('',*,*,#7182,.T.);
#9270=ORIENTED_EDGE('',*,*,#7183,.T.);
#9271=ORIENTED_EDGE('',*,*,#7155,.T.);
#9272=ORIENTED_EDGE('',*,*,#7183,.F.);
#9273=ORIENTED_EDGE('',*,*,#7182,.F.);
#9274=ORIENTED_EDGE('',*,*,#7184,.T.);
#9275=ORIENTED_EDGE('',*,*,#7185,.T.);
#9276=ORIENTED_EDGE('',*,*,#7184,.F.);
#9277=ORIENTED_EDGE('',*,*,#7186,.T.);
#9278=ORIENTED_EDGE('',*,*,#7187,.T.);
#9279=ORIENTED_EDGE('',*,*,#7167,.T.);
#9280=ORIENTED_EDGE('',*,*,#7187,.F.);
#9281=ORIENTED_EDGE('',*,*,#7186,.F.);
#9282=ORIENTED_EDGE('',*,*,#7188,.T.);
#9283=ORIENTED_EDGE('',*,*,#7189,.T.);
#9284=ORIENTED_EDGE('',*,*,#7188,.F.);
#9285=ORIENTED_EDGE('',*,*,#7190,.T.);
#9286=ORIENTED_EDGE('',*,*,#7157,.T.);
#9287=ORIENTED_EDGE('',*,*,#7191,.T.);
#9288=ORIENTED_EDGE('',*,*,#7192,.T.);
#9289=ORIENTED_EDGE('',*,*,#7192,.F.);
#9290=ORIENTED_EDGE('',*,*,#7193,.F.);
#9291=ORIENTED_EDGE('',*,*,#7194,.F.);
#9292=ORIENTED_EDGE('',*,*,#7195,.T.);
#9293=ORIENTED_EDGE('',*,*,#7196,.F.);
#9294=ORIENTED_EDGE('',*,*,#7197,.F.);
#9295=ORIENTED_EDGE('',*,*,#7198,.F.);
#9296=ORIENTED_EDGE('',*,*,#7195,.F.);
#9297=ORIENTED_EDGE('',*,*,#7199,.F.);
#9298=ORIENTED_EDGE('',*,*,#7189,.F.);
#9299=ORIENTED_EDGE('',*,*,#7200,.F.);
#9300=ORIENTED_EDGE('',*,*,#7185,.F.);
#9301=ORIENTED_EDGE('',*,*,#7201,.F.);
#9302=ORIENTED_EDGE('',*,*,#7181,.F.);
#9303=ORIENTED_EDGE('',*,*,#7202,.F.);
#9304=ORIENTED_EDGE('',*,*,#7203,.F.);
#9305=ORIENTED_EDGE('',*,*,#7204,.T.);
#9306=ORIENTED_EDGE('',*,*,#7205,.F.);
#9307=ORIENTED_EDGE('',*,*,#7206,.F.);
#9308=ORIENTED_EDGE('',*,*,#7207,.F.);
#9309=ORIENTED_EDGE('',*,*,#7204,.F.);
#9310=ORIENTED_EDGE('',*,*,#7208,.F.);
#9311=ORIENTED_EDGE('',*,*,#7178,.F.);
#9312=ORIENTED_EDGE('',*,*,#7209,.F.);
#9313=ORIENTED_EDGE('',*,*,#7174,.F.);
#9314=ORIENTED_EDGE('',*,*,#7210,.F.);
#9315=ORIENTED_EDGE('',*,*,#7211,.F.);
#9316=ORIENTED_EDGE('',*,*,#7212,.T.);
#9317=ORIENTED_EDGE('',*,*,#7213,.F.);
#9318=ORIENTED_EDGE('',*,*,#7214,.F.);
#9319=ORIENTED_EDGE('',*,*,#7215,.F.);
#9320=ORIENTED_EDGE('',*,*,#7212,.F.);
#9321=ORIENTED_EDGE('',*,*,#7216,.F.);
#9322=ORIENTED_EDGE('',*,*,#7171,.F.);
#9323=ORIENTED_EDGE('',*,*,#7217,.F.);
#9324=ORIENTED_EDGE('',*,*,#7148,.F.);
#9325=ORIENTED_EDGE('',*,*,#7218,.F.);
#9326=ORIENTED_EDGE('',*,*,#7219,.F.);
#9327=ORIENTED_EDGE('',*,*,#7220,.T.);
#9328=ORIENTED_EDGE('',*,*,#7221,.F.);
#9329=ORIENTED_EDGE('',*,*,#7222,.F.);
#9330=ORIENTED_EDGE('',*,*,#7223,.F.);
#9331=ORIENTED_EDGE('',*,*,#7220,.F.);
#9332=ORIENTED_EDGE('',*,*,#7224,.F.);
#9333=ORIENTED_EDGE('',*,*,#7191,.F.);
#9334=ORIENTED_EDGE('',*,*,#7158,.T.);
#9335=ORIENTED_EDGE('',*,*,#7190,.F.);
#9336=ORIENTED_EDGE('',*,*,#7197,.T.);
#9337=ORIENTED_EDGE('',*,*,#7225,.T.);
#9338=ORIENTED_EDGE('',*,*,#7226,.T.);
#9339=ORIENTED_EDGE('',*,*,#7193,.T.);
#9340=ORIENTED_EDGE('',*,*,#7180,.F.);
#9341=ORIENTED_EDGE('',*,*,#7163,.T.);
#9342=ORIENTED_EDGE('',*,*,#7179,.F.);
#9343=ORIENTED_EDGE('',*,*,#7206,.T.);
#9344=ORIENTED_EDGE('',*,*,#7227,.T.);
#9345=ORIENTED_EDGE('',*,*,#7228,.T.);
#9346=ORIENTED_EDGE('',*,*,#7202,.T.);
#9347=ORIENTED_EDGE('',*,*,#7173,.F.);
#9348=ORIENTED_EDGE('',*,*,#7165,.T.);
#9349=ORIENTED_EDGE('',*,*,#7172,.F.);
#9350=ORIENTED_EDGE('',*,*,#7214,.T.);
#9351=ORIENTED_EDGE('',*,*,#7229,.T.);
#9352=ORIENTED_EDGE('',*,*,#7230,.T.);
#9353=ORIENTED_EDGE('',*,*,#7210,.T.);
#9354=ORIENTED_EDGE('',*,*,#7147,.F.);
#9355=ORIENTED_EDGE('',*,*,#7159,.T.);
#9356=ORIENTED_EDGE('',*,*,#7145,.F.);
#9357=ORIENTED_EDGE('',*,*,#7222,.T.);
#9358=ORIENTED_EDGE('',*,*,#7231,.T.);
#9359=ORIENTED_EDGE('',*,*,#7232,.T.);
#9360=ORIENTED_EDGE('',*,*,#7218,.T.);
#9361=ORIENTED_EDGE('',*,*,#7199,.T.);
#9362=ORIENTED_EDGE('',*,*,#7233,.T.);
#9363=ORIENTED_EDGE('',*,*,#7234,.F.);
#9364=ORIENTED_EDGE('',*,*,#7233,.F.);
#9365=ORIENTED_EDGE('',*,*,#7200,.T.);
#9366=ORIENTED_EDGE('',*,*,#7235,.T.);
#9367=ORIENTED_EDGE('',*,*,#7236,.F.);
#9368=ORIENTED_EDGE('',*,*,#7235,.F.);
#9369=ORIENTED_EDGE('',*,*,#7201,.T.);
#9370=ORIENTED_EDGE('',*,*,#7237,.T.);
#9371=ORIENTED_EDGE('',*,*,#7238,.F.);
#9372=ORIENTED_EDGE('',*,*,#7237,.F.);
#9373=ORIENTED_EDGE('',*,*,#7208,.T.);
#9374=ORIENTED_EDGE('',*,*,#7239,.T.);
#9375=ORIENTED_EDGE('',*,*,#7240,.F.);
#9376=ORIENTED_EDGE('',*,*,#7239,.F.);
#9377=ORIENTED_EDGE('',*,*,#7209,.T.);
#9378=ORIENTED_EDGE('',*,*,#7241,.T.);
#9379=ORIENTED_EDGE('',*,*,#7242,.F.);
#9380=ORIENTED_EDGE('',*,*,#7241,.F.);
#9381=ORIENTED_EDGE('',*,*,#7216,.T.);
#9382=ORIENTED_EDGE('',*,*,#7243,.T.);
#9383=ORIENTED_EDGE('',*,*,#7244,.F.);
#9384=ORIENTED_EDGE('',*,*,#7243,.F.);
#9385=ORIENTED_EDGE('',*,*,#7217,.T.);
#9386=ORIENTED_EDGE('',*,*,#7245,.T.);
#9387=ORIENTED_EDGE('',*,*,#7246,.F.);
#9388=ORIENTED_EDGE('',*,*,#7245,.F.);
#9389=ORIENTED_EDGE('',*,*,#7224,.T.);
#9390=ORIENTED_EDGE('',*,*,#7247,.T.);
#9391=ORIENTED_EDGE('',*,*,#7248,.F.);
#9392=ORIENTED_EDGE('',*,*,#7247,.F.);
#9393=ORIENTED_EDGE('',*,*,#7249,.T.);
#9394=ORIENTED_EDGE('',*,*,#7250,.T.);
#9395=ORIENTED_EDGE('',*,*,#7166,.T.);
#9396=ORIENTED_EDGE('',*,*,#7250,.F.);
#9397=ORIENTED_EDGE('',*,*,#7249,.F.);
#9398=ORIENTED_EDGE('',*,*,#7251,.T.);
#9399=ORIENTED_EDGE('',*,*,#7252,.T.);
#9400=ORIENTED_EDGE('',*,*,#7251,.F.);
#9401=ORIENTED_EDGE('',*,*,#7253,.T.);
#9402=ORIENTED_EDGE('',*,*,#7254,.T.);
#9403=ORIENTED_EDGE('',*,*,#7156,.T.);
#9404=ORIENTED_EDGE('',*,*,#7254,.F.);
#9405=ORIENTED_EDGE('',*,*,#7253,.F.);
#9406=ORIENTED_EDGE('',*,*,#7255,.T.);
#9407=ORIENTED_EDGE('',*,*,#7256,.T.);
#9408=ORIENTED_EDGE('',*,*,#7255,.F.);
#9409=ORIENTED_EDGE('',*,*,#7229,.F.);
#9410=ORIENTED_EDGE('',*,*,#7213,.T.);
#9411=ORIENTED_EDGE('',*,*,#7215,.T.);
#9412=ORIENTED_EDGE('',*,*,#7211,.T.);
#9413=ORIENTED_EDGE('',*,*,#7230,.F.);
#9414=ORIENTED_EDGE('',*,*,#7257,.T.);
#9415=ORIENTED_EDGE('',*,*,#7258,.T.);
#9416=ORIENTED_EDGE('',*,*,#7257,.F.);
#9417=ORIENTED_EDGE('',*,*,#7225,.F.);
#9418=ORIENTED_EDGE('',*,*,#7196,.T.);
#9419=ORIENTED_EDGE('',*,*,#7198,.T.);
#9420=ORIENTED_EDGE('',*,*,#7194,.T.);
#9421=ORIENTED_EDGE('',*,*,#7226,.F.);
#9422=ORIENTED_EDGE('',*,*,#7259,.T.);
#9423=ORIENTED_EDGE('',*,*,#7260,.T.);
#9424=ORIENTED_EDGE('',*,*,#7259,.F.);
#9425=ORIENTED_EDGE('',*,*,#7227,.F.);
#9426=ORIENTED_EDGE('',*,*,#7205,.T.);
#9427=ORIENTED_EDGE('',*,*,#7207,.T.);
#9428=ORIENTED_EDGE('',*,*,#7203,.T.);
#9429=ORIENTED_EDGE('',*,*,#7228,.F.);
#9430=ORIENTED_EDGE('',*,*,#7261,.T.);
#9431=ORIENTED_EDGE('',*,*,#7262,.T.);
#9432=ORIENTED_EDGE('',*,*,#7261,.F.);
#9433=ORIENTED_EDGE('',*,*,#7231,.F.);
#9434=ORIENTED_EDGE('',*,*,#7221,.T.);
#9435=ORIENTED_EDGE('',*,*,#7223,.T.);
#9436=ORIENTED_EDGE('',*,*,#7219,.T.);
#9437=ORIENTED_EDGE('',*,*,#7232,.F.);
#9438=ORIENTED_EDGE('',*,*,#7263,.T.);
#9439=ORIENTED_EDGE('',*,*,#7264,.T.);
#9440=ORIENTED_EDGE('',*,*,#7263,.F.);
#9441=ORIENTED_EDGE('',*,*,#7265,.T.);
#9442=ORIENTED_EDGE('',*,*,#7266,.T.);
#9443=ORIENTED_EDGE('',*,*,#7161,.T.);
#9444=ORIENTED_EDGE('',*,*,#7266,.F.);
#9445=ORIENTED_EDGE('',*,*,#7265,.F.);
#9446=ORIENTED_EDGE('',*,*,#7267,.T.);
#9447=ORIENTED_EDGE('',*,*,#7268,.T.);
#9448=ORIENTED_EDGE('',*,*,#7267,.F.);
#9449=ORIENTED_EDGE('',*,*,#7269,.T.);
#9450=ORIENTED_EDGE('',*,*,#7270,.T.);
#9451=ORIENTED_EDGE('',*,*,#7160,.T.);
#9452=ORIENTED_EDGE('',*,*,#7270,.F.);
#9453=ORIENTED_EDGE('',*,*,#7269,.F.);
#9454=ORIENTED_EDGE('',*,*,#7271,.T.);
#9455=ORIENTED_EDGE('',*,*,#7272,.T.);
#9456=ORIENTED_EDGE('',*,*,#7271,.F.);
#9457=ORIENTED_EDGE('',*,*,#7273,.T.);
#9458=ORIENTED_EDGE('',*,*,#7252,.F.);
#9459=ORIENTED_EDGE('',*,*,#7273,.F.);
#9460=ORIENTED_EDGE('',*,*,#7274,.T.);
#9461=ORIENTED_EDGE('',*,*,#7272,.F.);
#9462=ORIENTED_EDGE('',*,*,#7274,.F.);
#9463=ORIENTED_EDGE('',*,*,#7275,.T.);
#9464=ORIENTED_EDGE('',*,*,#7256,.F.);
#9465=ORIENTED_EDGE('',*,*,#7275,.F.);
#9466=ORIENTED_EDGE('',*,*,#7276,.T.);
#9467=ORIENTED_EDGE('',*,*,#7268,.F.);
#9468=ORIENTED_EDGE('',*,*,#7276,.F.);
#9469=ORIENTED_EDGE('',*,*,#7277,.T.);
#9470=ORIENTED_EDGE('',*,*,#7264,.F.);
#9471=ORIENTED_EDGE('',*,*,#7277,.F.);
#9472=ORIENTED_EDGE('',*,*,#7278,.T.);
#9473=ORIENTED_EDGE('',*,*,#7260,.F.);
#9474=ORIENTED_EDGE('',*,*,#7278,.F.);
#9475=ORIENTED_EDGE('',*,*,#7279,.T.);
#9476=ORIENTED_EDGE('',*,*,#7262,.F.);
#9477=ORIENTED_EDGE('',*,*,#7279,.F.);
#9478=ORIENTED_EDGE('',*,*,#7280,.T.);
#9479=ORIENTED_EDGE('',*,*,#7258,.F.);
#9480=ORIENTED_EDGE('',*,*,#7280,.F.);
#9481=ORIENTED_EDGE('',*,*,#7149,.T.);
#9482=ORIENTED_EDGE('',*,*,#7281,.T.);
#9483=ORIENTED_EDGE('',*,*,#7282,.T.);
#9484=ORIENTED_EDGE('',*,*,#7283,.F.);
#9485=ORIENTED_EDGE('',*,*,#7152,.T.);
#9486=ORIENTED_EDGE('',*,*,#7284,.T.);
#9487=ORIENTED_EDGE('',*,*,#7285,.T.);
#9488=ORIENTED_EDGE('',*,*,#7281,.F.);
#9489=ORIENTED_EDGE('',*,*,#7151,.T.);
#9490=ORIENTED_EDGE('',*,*,#7286,.T.);
#9491=ORIENTED_EDGE('',*,*,#7287,.T.);
#9492=ORIENTED_EDGE('',*,*,#7284,.F.);
#9493=ORIENTED_EDGE('',*,*,#7288,.T.);
#9494=ORIENTED_EDGE('',*,*,#7286,.F.);
#9495=ORIENTED_EDGE('',*,*,#7150,.T.);
#9496=ORIENTED_EDGE('',*,*,#7283,.T.);
#9497=ORIENTED_EDGE('',*,*,#7288,.F.);
#9498=ORIENTED_EDGE('',*,*,#7289,.F.);
#9499=ORIENTED_EDGE('',*,*,#7290,.F.);
#9500=ORIENTED_EDGE('',*,*,#7291,.T.);
#9501=ORIENTED_EDGE('',*,*,#7282,.F.);
#9502=ORIENTED_EDGE('',*,*,#7292,.F.);
#9503=ORIENTED_EDGE('',*,*,#7293,.F.);
#9504=ORIENTED_EDGE('',*,*,#7289,.T.);
#9505=ORIENTED_EDGE('',*,*,#7287,.F.);
#9506=ORIENTED_EDGE('',*,*,#7291,.F.);
#9507=ORIENTED_EDGE('',*,*,#7294,.F.);
#9508=ORIENTED_EDGE('',*,*,#7295,.T.);
#9509=ORIENTED_EDGE('',*,*,#7285,.F.);
#9510=ORIENTED_EDGE('',*,*,#7295,.F.);
#9511=ORIENTED_EDGE('',*,*,#7296,.F.);
#9512=ORIENTED_EDGE('',*,*,#7292,.T.);
#9513=ORIENTED_EDGE('',*,*,#7296,.T.);
#9514=ORIENTED_EDGE('',*,*,#7294,.T.);
#9515=ORIENTED_EDGE('',*,*,#7290,.T.);
#9516=ORIENTED_EDGE('',*,*,#7293,.T.);
#9517=ORIENTED_EDGE('',*,*,#7248,.T.);
#9518=ORIENTED_EDGE('',*,*,#7246,.T.);
#9519=ORIENTED_EDGE('',*,*,#7244,.T.);
#9520=ORIENTED_EDGE('',*,*,#7242,.T.);
#9521=ORIENTED_EDGE('',*,*,#7240,.T.);
#9522=ORIENTED_EDGE('',*,*,#7238,.T.);
#9523=ORIENTED_EDGE('',*,*,#7236,.T.);
#9524=ORIENTED_EDGE('',*,*,#7234,.T.);
#12883=CYLINDRICAL_SURFACE('',#13876,4.25000000000001);
#12884=CYLINDRICAL_SURFACE('',#13882,4.25);
#12885=CYLINDRICAL_SURFACE('',#13888,4.25);
#12886=CYLINDRICAL_SURFACE('',#13892,4.25000000000001);
#12887=CYLINDRICAL_SURFACE('',#13896,4.25000000000001);
#12888=CYLINDRICAL_SURFACE('',#13905,4.25);
#12889=CYLINDRICAL_SURFACE('',#13912,4.25);
#12890=CYLINDRICAL_SURFACE('',#13919,4.25000000000001);
#12891=CYLINDRICAL_SURFACE('',#13936,2.6);
#12892=CYLINDRICAL_SURFACE('',#13938,2.6);
#12893=CYLINDRICAL_SURFACE('',#13940,2.6);
#12894=CYLINDRICAL_SURFACE('',#13942,2.6);
#12895=CYLINDRICAL_SURFACE('',#13944,2.6);
#12896=CYLINDRICAL_SURFACE('',#13946,2.6);
#12897=CYLINDRICAL_SURFACE('',#13948,2.6);
#12898=CYLINDRICAL_SURFACE('',#13950,2.6);
#12899=CYLINDRICAL_SURFACE('',#13954,3.225);
#12900=CYLINDRICAL_SURFACE('',#13958,3.225);
#12901=CYLINDRICAL_SURFACE('',#13960,3.225);
#12902=CYLINDRICAL_SURFACE('',#13962,3.225);
#12903=CYLINDRICAL_SURFACE('',#13964,3.225);
#12904=CYLINDRICAL_SURFACE('',#13966,3.225);
#12905=CYLINDRICAL_SURFACE('',#13970,3.225);
#12906=CYLINDRICAL_SURFACE('',#13974,3.225);
#13041=ADVANCED_FACE('',(#2081),#1057,.F.);
#13042=ADVANCED_FACE('',(#2082,#1514,#1515,#1516,#1517,#1518,#1519,#1520,
#1521,#1522,#1523,#1524,#1525),#1593,.T.);
#13043=ADVANCED_FACE('',(#2083),#1058,.F.);
#13044=ADVANCED_FACE('',(#2084),#12883,.F.);
#13045=ADVANCED_FACE('',(#2085),#1059,.F.);
#13046=ADVANCED_FACE('',(#2086),#1060,.F.);
#13047=ADVANCED_FACE('',(#2087),#12884,.F.);
#13048=ADVANCED_FACE('',(#2088),#1061,.F.);
#13049=ADVANCED_FACE('',(#2089),#1062,.F.);
#13050=ADVANCED_FACE('',(#2090),#12885,.F.);
#13051=ADVANCED_FACE('',(#2091),#1063,.F.);
#13052=ADVANCED_FACE('',(#2092),#12886,.F.);
#13053=ADVANCED_FACE('',(#2093),#1064,.F.);
#13054=ADVANCED_FACE('',(#2094),#12887,.F.);
#13055=ADVANCED_FACE('',(#2095,#1526),#1594,.T.);
#13056=ADVANCED_FACE('',(#2096,#1527),#1595,.T.);
#13057=ADVANCED_FACE('',(#2097,#1528),#1596,.T.);
#13058=ADVANCED_FACE('',(#2098),#12888,.F.);
#13059=ADVANCED_FACE('',(#2099,#1529),#1597,.T.);
#13060=ADVANCED_FACE('',(#2100,#1530),#1598,.T.);
#13061=ADVANCED_FACE('',(#2101),#12889,.F.);
#13062=ADVANCED_FACE('',(#2102,#1531),#1599,.T.);
#13063=ADVANCED_FACE('',(#2103,#1532),#1600,.T.);
#13064=ADVANCED_FACE('',(#2104),#12890,.F.);
#13065=ADVANCED_FACE('',(#2105,#1533),#1601,.T.);
#13066=ADVANCED_FACE('',(#2106),#1065,.F.);
#13067=ADVANCED_FACE('',(#2107),#1066,.F.);
#13068=ADVANCED_FACE('',(#2108),#1067,.F.);
#13069=ADVANCED_FACE('',(#2109),#1068,.F.);
#13070=ADVANCED_FACE('',(#2110),#12891,.F.);
#13071=ADVANCED_FACE('',(#2111),#12892,.F.);
#13072=ADVANCED_FACE('',(#2112),#12893,.F.);
#13073=ADVANCED_FACE('',(#2113),#12894,.F.);
#13074=ADVANCED_FACE('',(#2114),#12895,.F.);
#13075=ADVANCED_FACE('',(#2115),#12896,.F.);
#13076=ADVANCED_FACE('',(#2116),#12897,.F.);
#13077=ADVANCED_FACE('',(#2117),#12898,.F.);
#13078=ADVANCED_FACE('',(#2118),#1069,.F.);
#13079=ADVANCED_FACE('',(#2119),#12899,.F.);
#13080=ADVANCED_FACE('',(#2120),#1070,.F.);
#13081=ADVANCED_FACE('',(#2121),#12900,.F.);
#13082=ADVANCED_FACE('',(#2122),#12901,.F.);
#13083=ADVANCED_FACE('',(#2123),#12902,.F.);
#13084=ADVANCED_FACE('',(#2124),#12903,.F.);
#13085=ADVANCED_FACE('',(#2125),#12904,.F.);
#13086=ADVANCED_FACE('',(#2126),#1071,.F.);
#13087=ADVANCED_FACE('',(#2127),#12905,.F.);
#13088=ADVANCED_FACE('',(#2128),#1072,.F.);
#13089=ADVANCED_FACE('',(#2129),#12906,.F.);
#13090=ADVANCED_FACE('',(#2130),#1073,.F.);
#13091=ADVANCED_FACE('',(#2131),#1074,.F.);
#13092=ADVANCED_FACE('',(#2132),#1075,.F.);
#13093=ADVANCED_FACE('',(#2133),#1076,.F.);
#13094=ADVANCED_FACE('',(#2134),#1077,.F.);
#13095=ADVANCED_FACE('',(#2135),#1078,.F.);
#13096=ADVANCED_FACE('',(#2136),#1079,.F.);
#13097=ADVANCED_FACE('',(#2137),#1080,.F.);
#13098=ADVANCED_FACE('',(#2138),#1602,.T.);
#13099=ADVANCED_FACE('',(#2139),#1603,.T.);
#13100=ADVANCED_FACE('',(#2140),#1604,.T.);
#13101=ADVANCED_FACE('',(#2141),#1605,.T.);
#13102=ADVANCED_FACE('',(#2142),#1606,.T.);
#13103=ADVANCED_FACE('',(#2143),#1607,.T.);
#13104=ADVANCED_FACE('',(#2144),#1608,.T.);
#13105=ADVANCED_FACE('',(#2145),#1609,.T.);
#13106=ADVANCED_FACE('',(#2146,#1534,#1535,#1536,#1537,#1538,#1539,#1540,
#1541),#1610,.F.);
#13636=CLOSED_SHELL('',(#13041,#13042,#13043,#13044,#13045,#13046,#13047,
#13048,#13049,#13050,#13051,#13052,#13053,#13054,#13055,#13056,#13057,#13058,
#13059,#13060,#13061,#13062,#13063,#13064,#13065,#13066,#13067,#13068,#13069,
#13070,#13071,#13072,#13073,#13074,#13075,#13076,#13077,#13078,#13079,#13080,
#13081,#13082,#13083,#13084,#13085,#13086,#13087,#13088,#13089,#13090,#13091,
#13092,#13093,#13094,#13095,#13096,#13097,#13098,#13099,#13100,#13101,#13102,
#13103,#13104,#13105,#13106));
#13854=AXIS2_PLACEMENT_3D('',#19002,#15313,#15314);
#13855=AXIS2_PLACEMENT_3D('',#19003,#15315,#15316);
#13856=AXIS2_PLACEMENT_3D('',#19013,#15317,#15318);
#13857=AXIS2_PLACEMENT_3D('',#19021,#15319,#15320);
#13858=AXIS2_PLACEMENT_3D('',#19022,#15321,#15322);
#13859=AXIS2_PLACEMENT_3D('',#19032,#15327,#15328);
#13860=AXIS2_PLACEMENT_3D('',#19034,#15329,#15330);
#13861=AXIS2_PLACEMENT_3D('',#19036,#15331,#15332);
#13862=AXIS2_PLACEMENT_3D('',#19038,#15333,#15334);
#13863=AXIS2_PLACEMENT_3D('',#19041,#15335,#15336);
#13864=AXIS2_PLACEMENT_3D('',#19042,#15337,#15338);
#13865=AXIS2_PLACEMENT_3D('',#19043,#15339,#15340);
#13866=AXIS2_PLACEMENT_3D('',#19045,#15341,#15342);
#13867=AXIS2_PLACEMENT_3D('',#19047,#15343,#15344);
#13868=AXIS2_PLACEMENT_3D('',#19050,#15345,#15346);
#13869=AXIS2_PLACEMENT_3D('',#19051,#15347,#15348);
#13870=AXIS2_PLACEMENT_3D('',#19054,#15349,#15350);
#13871=AXIS2_PLACEMENT_3D('',#19055,#15351,#15352);
#13872=AXIS2_PLACEMENT_3D('',#19057,#15353,#15354);
#13873=AXIS2_PLACEMENT_3D('',#19059,#15355,#15356);
#13874=AXIS2_PLACEMENT_3D('',#19060,#15357,#15358);
#13875=AXIS2_PLACEMENT_3D('',#19062,#15359,#15360);
#13876=AXIS2_PLACEMENT_3D('',#19064,#15362,#15363);
#13877=AXIS2_PLACEMENT_3D('',#19067,#15365,#15366);
#13878=AXIS2_PLACEMENT_3D('',#19068,#15367,#15368);
#13879=AXIS2_PLACEMENT_3D('',#19083,#15369,#15370);
#13880=AXIS2_PLACEMENT_3D('',#19084,#15371,#15372);
#13881=AXIS2_PLACEMENT_3D('',#19086,#15373,#15374);
#13882=AXIS2_PLACEMENT_3D('',#19088,#15376,#15377);
#13883=AXIS2_PLACEMENT_3D('',#19091,#15379,#15380);
#13884=AXIS2_PLACEMENT_3D('',#19092,#15381,#15382);
#13885=AXIS2_PLACEMENT_3D('',#19107,#15383,#15384);
#13886=AXIS2_PLACEMENT_3D('',#19108,#15385,#15386);
#13887=AXIS2_PLACEMENT_3D('',#19110,#15387,#15388);
#13888=AXIS2_PLACEMENT_3D('',#19112,#15390,#15391);
#13889=AXIS2_PLACEMENT_3D('',#19115,#15393,#15394);
#13890=AXIS2_PLACEMENT_3D('',#19116,#15395,#15396);
#13891=AXIS2_PLACEMENT_3D('',#19118,#15397,#15398);
#13892=AXIS2_PLACEMENT_3D('',#19120,#15400,#15401);
#13893=AXIS2_PLACEMENT_3D('',#19123,#15403,#15404);
#13894=AXIS2_PLACEMENT_3D('',#19124,#15405,#15406);
#13895=AXIS2_PLACEMENT_3D('',#19139,#15407,#15408);
#13896=AXIS2_PLACEMENT_3D('',#19140,#15409,#15410);
#13897=AXIS2_PLACEMENT_3D('',#19149,#15412,#15413);
#13898=AXIS2_PLACEMENT_3D('',#19156,#15415,#15416);
#13899=AXIS2_PLACEMENT_3D('',#19157,#15417,#15418);
#13900=AXIS2_PLACEMENT_3D('',#19159,#15419,#15420);
#13901=AXIS2_PLACEMENT_3D('',#19160,#15421,#15422);
#13902=AXIS2_PLACEMENT_3D('',#19162,#15423,#15424);
#13903=AXIS2_PLACEMENT_3D('',#19163,#15425,#15426);
#13904=AXIS2_PLACEMENT_3D('',#19165,#15427,#15428);
#13905=AXIS2_PLACEMENT_3D('',#19166,#15429,#15430);
#13906=AXIS2_PLACEMENT_3D('',#19175,#15432,#15433);
#13907=AXIS2_PLACEMENT_3D('',#19182,#15435,#15436);
#13908=AXIS2_PLACEMENT_3D('',#19183,#15437,#15438);
#13909=AXIS2_PLACEMENT_3D('',#19185,#15439,#15440);
#13910=AXIS2_PLACEMENT_3D('',#19186,#15441,#15442);
#13911=AXIS2_PLACEMENT_3D('',#19188,#15443,#15444);
#13912=AXIS2_PLACEMENT_3D('',#19189,#15445,#15446);
#13913=AXIS2_PLACEMENT_3D('',#19198,#15448,#15449);
#13914=AXIS2_PLACEMENT_3D('',#19205,#15451,#15452);
#13915=AXIS2_PLACEMENT_3D('',#19206,#15453,#15454);
#13916=AXIS2_PLACEMENT_3D('',#19208,#15455,#15456);
#13917=AXIS2_PLACEMENT_3D('',#19209,#15457,#15458);
#13918=AXIS2_PLACEMENT_3D('',#19211,#15459,#15460);
#13919=AXIS2_PLACEMENT_3D('',#19212,#15461,#15462);
#13920=AXIS2_PLACEMENT_3D('',#19221,#15464,#15465);
#13921=AXIS2_PLACEMENT_3D('',#19228,#15467,#15468);
#13922=AXIS2_PLACEMENT_3D('',#19229,#15469,#15470);
#13923=AXIS2_PLACEMENT_3D('',#19231,#15471,#15472);
#13924=AXIS2_PLACEMENT_3D('',#19232,#15473,#15474);
#13925=AXIS2_PLACEMENT_3D('',#19234,#15475,#15476);
#13926=AXIS2_PLACEMENT_3D('',#19235,#15477,#15478);
#13927=AXIS2_PLACEMENT_3D('',#19236,#15479,#15480);
#13928=AXIS2_PLACEMENT_3D('',#19238,#15481,#15482);
#13929=AXIS2_PLACEMENT_3D('',#19239,#15483,#15484);
#13930=AXIS2_PLACEMENT_3D('',#19240,#15485,#15486);
#13931=AXIS2_PLACEMENT_3D('',#19242,#15487,#15488);
#13932=AXIS2_PLACEMENT_3D('',#19243,#15489,#15490);
#13933=AXIS2_PLACEMENT_3D('',#19244,#15491,#15492);
#13934=AXIS2_PLACEMENT_3D('',#19246,#15493,#15494);
#13935=AXIS2_PLACEMENT_3D('',#19247,#15495,#15496);
#13936=AXIS2_PLACEMENT_3D('',#19248,#15497,#15498);
#13937=AXIS2_PLACEMENT_3D('',#19251,#15500,#15501);
#13938=AXIS2_PLACEMENT_3D('',#19252,#15502,#15503);
#13939=AXIS2_PLACEMENT_3D('',#19255,#15505,#15506);
#13940=AXIS2_PLACEMENT_3D('',#19256,#15507,#15508);
#13941=AXIS2_PLACEMENT_3D('',#19259,#15510,#15511);
#13942=AXIS2_PLACEMENT_3D('',#19260,#15512,#15513);
#13943=AXIS2_PLACEMENT_3D('',#19263,#15515,#15516);
#13944=AXIS2_PLACEMENT_3D('',#19264,#15517,#15518);
#13945=AXIS2_PLACEMENT_3D('',#19267,#15520,#15521);
#13946=AXIS2_PLACEMENT_3D('',#19268,#15522,#15523);
#13947=AXIS2_PLACEMENT_3D('',#19271,#15525,#15526);
#13948=AXIS2_PLACEMENT_3D('',#19272,#15527,#15528);
#13949=AXIS2_PLACEMENT_3D('',#19275,#15530,#15531);
#13950=AXIS2_PLACEMENT_3D('',#19276,#15532,#15533);
#13951=AXIS2_PLACEMENT_3D('',#19279,#15535,#15536);
#13952=AXIS2_PLACEMENT_3D('',#19280,#15537,#15538);
#13953=AXIS2_PLACEMENT_3D('',#19282,#15539,#15540);
#13954=AXIS2_PLACEMENT_3D('',#19284,#15542,#15543);
#13955=AXIS2_PLACEMENT_3D('',#19287,#15545,#15546);
#13956=AXIS2_PLACEMENT_3D('',#19288,#15547,#15548);
#13957=AXIS2_PLACEMENT_3D('',#19290,#15549,#15550);
#13958=AXIS2_PLACEMENT_3D('',#19292,#15552,#15553);
#13959=AXIS2_PLACEMENT_3D('',#19295,#15555,#15556);
#13960=AXIS2_PLACEMENT_3D('',#19296,#15557,#15558);
#13961=AXIS2_PLACEMENT_3D('',#19299,#15560,#15561);
#13962=AXIS2_PLACEMENT_3D('',#19300,#15562,#15563);
#13963=AXIS2_PLACEMENT_3D('',#19303,#15565,#15566);
#13964=AXIS2_PLACEMENT_3D('',#19304,#15567,#15568);
#13965=AXIS2_PLACEMENT_3D('',#19307,#15570,#15571);
#13966=AXIS2_PLACEMENT_3D('',#19308,#15572,#15573);
#13967=AXIS2_PLACEMENT_3D('',#19311,#15575,#15576);
#13968=AXIS2_PLACEMENT_3D('',#19312,#15577,#15578);
#13969=AXIS2_PLACEMENT_3D('',#19314,#15579,#15580);
#13970=AXIS2_PLACEMENT_3D('',#19316,#15582,#15583);
#13971=AXIS2_PLACEMENT_3D('',#19319,#15585,#15586);
#13972=AXIS2_PLACEMENT_3D('',#19320,#15587,#15588);
#13973=AXIS2_PLACEMENT_3D('',#19322,#15589,#15590);
#13974=AXIS2_PLACEMENT_3D('',#19324,#15592,#15593);
#13975=AXIS2_PLACEMENT_3D('',#19327,#15595,#15596);
#13976=AXIS2_PLACEMENT_3D('',#19328,#15597,#15598);
#13977=AXIS2_PLACEMENT_3D('',#19331,#15600,#15601);
#13978=AXIS2_PLACEMENT_3D('',#19334,#15603,#15604);
#13979=AXIS2_PLACEMENT_3D('',#19337,#15606,#15607);
#13980=AXIS2_PLACEMENT_3D('',#19340,#15609,#15610);
#13981=AXIS2_PLACEMENT_3D('',#19343,#15612,#15613);
#13982=AXIS2_PLACEMENT_3D('',#19346,#15615,#15616);
#13983=AXIS2_PLACEMENT_3D('',#19349,#15618,#15619);
#13984=AXIS2_PLACEMENT_3D('',#19352,#15621,#15622);
#13985=AXIS2_PLACEMENT_3D('',#19358,#15626,#15627);
#13986=AXIS2_PLACEMENT_3D('',#19362,#15630,#15631);
#13987=AXIS2_PLACEMENT_3D('',#19366,#15634,#15635);
#13988=AXIS2_PLACEMENT_3D('',#19368,#15637,#15638);
#13989=AXIS2_PLACEMENT_3D('',#19374,#15642,#15643);
#13990=AXIS2_PLACEMENT_3D('',#19378,#15646,#15647);
#13991=AXIS2_PLACEMENT_3D('',#19382,#15650,#15651);
#13992=AXIS2_PLACEMENT_3D('',#19384,#15653,#15654);
#15313=DIRECTION('axis',(0.,0.,1.));
#15314=DIRECTION('refdir',(1.,0.,0.));
#15315=DIRECTION('center_axis',(0.,1.,0.));
#15316=DIRECTION('ref_axis',(-0.429672959082026,0.,0.902984578070797));
#15317=DIRECTION('center_axis',(0.,1.,0.));
#15318=DIRECTION('ref_axis',(-1.,0.,0.));
#15319=DIRECTION('center_axis',(0.,-1.,0.));
#15320=DIRECTION('ref_axis',(-1.,0.,0.));
#15321=DIRECTION('center_axis',(0.,1.,0.));
#15322=DIRECTION('ref_axis',(0.,0.,1.));
#15323=DIRECTION('',(0.,0.,1.));
#15324=DIRECTION('',(1.,0.,0.));
#15325=DIRECTION('',(0.,0.,-1.));
#15326=DIRECTION('',(-1.,0.,0.));
#15327=DIRECTION('center_axis',(0.,1.,0.));
#15328=DIRECTION('ref_axis',(1.,0.,0.));
#15329=DIRECTION('center_axis',(0.,1.,0.));
#15330=DIRECTION('ref_axis',(1.,0.,0.));
#15331=DIRECTION('center_axis',(0.,1.,0.));
#15332=DIRECTION('ref_axis',(1.,0.,0.));
#15333=DIRECTION('center_axis',(0.,1.,0.));
#15334=DIRECTION('ref_axis',(1.,0.,0.));
#15335=DIRECTION('center_axis',(0.,1.,0.));
#15336=DIRECTION('ref_axis',(-1.,0.,0.));
#15337=DIRECTION('center_axis',(0.,1.,0.));
#15338=DIRECTION('ref_axis',(1.,0.,0.));
#15339=DIRECTION('center_axis',(0.,1.,0.));
#15340=DIRECTION('ref_axis',(1.,0.,0.));
#15341=DIRECTION('center_axis',(0.,1.,0.));
#15342=DIRECTION('ref_axis',(1.,0.,0.));
#15343=DIRECTION('center_axis',(0.,1.,0.));
#15344=DIRECTION('ref_axis',(1.,0.,0.));
#15345=DIRECTION('center_axis',(0.,1.,0.));
#15346=DIRECTION('ref_axis',(1.,0.,0.));
#15347=DIRECTION('center_axis',(0.,1.,0.));
#15348=DIRECTION('ref_axis',(1.,0.,0.));
#15349=DIRECTION('center_axis',(0.,1.,0.));
#15350=DIRECTION('ref_axis',(1.,0.,0.));
#15351=DIRECTION('center_axis',(0.,1.,0.));
#15352=DIRECTION('ref_axis',(1.,0.,0.));
#15353=DIRECTION('center_axis',(0.,1.,0.));
#15354=DIRECTION('ref_axis',(1.,0.,0.));
#15355=DIRECTION('center_axis',(0.,1.,0.));
#15356=DIRECTION('ref_axis',(1.,0.,0.));
#15357=DIRECTION('center_axis',(0.,1.,0.));
#15358=DIRECTION('ref_axis',(1.,0.,0.));
#15359=DIRECTION('center_axis',(0.,-1.,0.));
#15360=DIRECTION('ref_axis',(1.,0.,0.));
#15361=DIRECTION('',(-0.707106781186537,0.707106781186558,8.65956056235481E-17));
#15362=DIRECTION('center_axis',(0.,-1.,0.));
#15363=DIRECTION('ref_axis',(1.,0.,0.));
#15364=DIRECTION('',(0.,-1.,0.));
#15365=DIRECTION('center_axis',(0.,-1.,0.));
#15366=DIRECTION('ref_axis',(1.,0.,0.));
#15367=DIRECTION('center_axis',(0.,1.,0.));
#15368=DIRECTION('ref_axis',(0.429672959082026,0.,-0.902984578070797));
#15369=DIRECTION('center_axis',(0.,-1.,0.));
#15370=DIRECTION('ref_axis',(1.,0.,0.));
#15371=DIRECTION('center_axis',(0.,1.,0.));
#15372=DIRECTION('ref_axis',(1.,0.,0.));
#15373=DIRECTION('center_axis',(0.,-1.,0.));
#15374=DIRECTION('ref_axis',(1.,0.,0.));
#15375=DIRECTION('',(-0.707106781186547,0.707106781186548,8.65956056235493E-17));
#15376=DIRECTION('center_axis',(0.,-1.,0.));
#15377=DIRECTION('ref_axis',(1.,0.,0.));
#15378=DIRECTION('',(0.,-1.,0.));
#15379=DIRECTION('center_axis',(0.,-1.,0.));
#15380=DIRECTION('ref_axis',(1.,0.,0.));
#15381=DIRECTION('center_axis',(0.,1.,0.));
#15382=DIRECTION('ref_axis',(0.429672959082009,0.,0.902984578070805));
#15383=DIRECTION('center_axis',(0.,-1.,0.));
#15384=DIRECTION('ref_axis',(1.,0.,0.));
#15385=DIRECTION('center_axis',(0.,1.,0.));
#15386=DIRECTION('ref_axis',(1.,0.,0.));
#15387=DIRECTION('center_axis',(0.,-1.,0.));
#15388=DIRECTION('ref_axis',(1.,0.,0.));
#15389=DIRECTION('',(-0.707106781186547,0.707106781186548,8.65956056235493E-17));
#15390=DIRECTION('center_axis',(0.,-1.,0.));
#15391=DIRECTION('ref_axis',(1.,0.,0.));
#15392=DIRECTION('',(0.,-1.,0.));
#15393=DIRECTION('center_axis',(0.,-1.,0.));
#15394=DIRECTION('ref_axis',(1.,0.,0.));
#15395=DIRECTION('center_axis',(0.,1.,0.));
#15396=DIRECTION('ref_axis',(1.,0.,0.));
#15397=DIRECTION('center_axis',(0.,-1.,0.));
#15398=DIRECTION('ref_axis',(1.,0.,0.));
#15399=DIRECTION('',(-0.707106781186537,0.707106781186558,8.65956056235481E-17));
#15400=DIRECTION('center_axis',(0.,-1.,0.));
#15401=DIRECTION('ref_axis',(1.,0.,0.));
#15402=DIRECTION('',(0.,-1.,0.));
#15403=DIRECTION('center_axis',(0.,-1.,0.));
#15404=DIRECTION('ref_axis',(1.,0.,0.));
#15405=DIRECTION('center_axis',(0.,1.,0.));
#15406=DIRECTION('ref_axis',(-0.429672959082014,0.,-0.902984578070803));
#15407=DIRECTION('center_axis',(0.,-1.,0.));
#15408=DIRECTION('ref_axis',(-1.,0.,0.));
#15409=DIRECTION('center_axis',(0.,-1.,0.));
#15410=DIRECTION('ref_axis',(-0.429672959082013,0.,-0.902984578070803));
#15411=DIRECTION('',(0.,1.,0.));
#15412=DIRECTION('center_axis',(0.,-1.,0.));
#15413=DIRECTION('ref_axis',(1.,0.,0.));
#15414=DIRECTION('',(0.,-1.,0.));
#15415=DIRECTION('center_axis',(0.,1.,0.));
#15416=DIRECTION('ref_axis',(1.,0.,0.));
#15417=DIRECTION('center_axis',(0.,1.,0.));
#15418=DIRECTION('ref_axis',(1.,0.,0.));
#15419=DIRECTION('center_axis',(0.,1.,0.));
#15420=DIRECTION('ref_axis',(1.,0.,0.));
#15421=DIRECTION('center_axis',(0.,1.,0.));
#15422=DIRECTION('ref_axis',(1.,0.,0.));
#15423=DIRECTION('center_axis',(0.,1.,0.));
#15424=DIRECTION('ref_axis',(1.,0.,0.));
#15425=DIRECTION('center_axis',(0.,1.,0.));
#15426=DIRECTION('ref_axis',(1.,0.,0.));
#15427=DIRECTION('center_axis',(0.,1.,0.));
#15428=DIRECTION('ref_axis',(1.,0.,0.));
#15429=DIRECTION('center_axis',(0.,-1.,0.));
#15430=DIRECTION('ref_axis',(0.429672959082017,0.,0.902984578070801));
#15431=DIRECTION('',(0.,1.,0.));
#15432=DIRECTION('center_axis',(0.,-1.,0.));
#15433=DIRECTION('ref_axis',(1.,0.,0.));
#15434=DIRECTION('',(0.,-1.,0.));
#15435=DIRECTION('center_axis',(0.,1.,0.));
#15436=DIRECTION('ref_axis',(1.,0.,0.));
#15437=DIRECTION('center_axis',(0.,1.,0.));
#15438=DIRECTION('ref_axis',(1.,0.,0.));
#15439=DIRECTION('center_axis',(0.,1.,0.));
#15440=DIRECTION('ref_axis',(1.,0.,0.));
#15441=DIRECTION('center_axis',(0.,1.,0.));
#15442=DIRECTION('ref_axis',(1.,0.,0.));
#15443=DIRECTION('center_axis',(0.,1.,0.));
#15444=DIRECTION('ref_axis',(1.,0.,0.));
#15445=DIRECTION('center_axis',(0.,-1.,0.));
#15446=DIRECTION('ref_axis',(0.429672959082017,0.,-0.902984578070801));
#15447=DIRECTION('',(0.,1.,0.));
#15448=DIRECTION('center_axis',(0.,-1.,0.));
#15449=DIRECTION('ref_axis',(1.,0.,0.));
#15450=DIRECTION('',(0.,-1.,0.));
#15451=DIRECTION('center_axis',(0.,1.,0.));
#15452=DIRECTION('ref_axis',(1.,0.,0.));
#15453=DIRECTION('center_axis',(0.,1.,0.));
#15454=DIRECTION('ref_axis',(1.,0.,0.));
#15455=DIRECTION('center_axis',(0.,1.,0.));
#15456=DIRECTION('ref_axis',(1.,0.,0.));
#15457=DIRECTION('center_axis',(0.,1.,0.));
#15458=DIRECTION('ref_axis',(1.,0.,0.));
#15459=DIRECTION('center_axis',(0.,1.,0.));
#15460=DIRECTION('ref_axis',(1.,0.,0.));
#15461=DIRECTION('center_axis',(0.,-1.,0.));
#15462=DIRECTION('ref_axis',(-0.429672959082013,0.,0.902984578070803));
#15463=DIRECTION('',(0.,1.,0.));
#15464=DIRECTION('center_axis',(0.,-1.,0.));
#15465=DIRECTION('ref_axis',(1.,0.,0.));
#15466=DIRECTION('',(0.,-1.,0.));
#15467=DIRECTION('center_axis',(0.,1.,0.));
#15468=DIRECTION('ref_axis',(1.,0.,0.));
#15469=DIRECTION('center_axis',(0.,1.,0.));
#15470=DIRECTION('ref_axis',(1.,0.,0.));
#15471=DIRECTION('center_axis',(0.,1.,0.));
#15472=DIRECTION('ref_axis',(1.,0.,0.));
#15473=DIRECTION('center_axis',(0.,1.,0.));
#15474=DIRECTION('ref_axis',(0.429672959082025,0.,0.902984578070798));
#15475=DIRECTION('center_axis',(0.,-1.,0.));
#15476=DIRECTION('ref_axis',(1.,0.,0.));
#15477=DIRECTION('center_axis',(0.,-1.,0.));
#15478=DIRECTION('ref_axis',(1.,0.,0.));
#15479=DIRECTION('center_axis',(0.,1.,0.));
#15480=DIRECTION('ref_axis',(-0.429672959082016,0.,-0.902984578070802));
#15481=DIRECTION('center_axis',(0.,-1.,0.));
#15482=DIRECTION('ref_axis',(1.,0.,0.));
#15483=DIRECTION('center_axis',(0.,-1.,0.));
#15484=DIRECTION('ref_axis',(1.,0.,0.));
#15485=DIRECTION('center_axis',(0.,1.,0.));
#15486=DIRECTION('ref_axis',(-0.429672959082016,0.,0.902984578070802));
#15487=DIRECTION('center_axis',(0.,-1.,0.));
#15488=DIRECTION('ref_axis',(1.,0.,0.));
#15489=DIRECTION('center_axis',(0.,-1.,0.));
#15490=DIRECTION('ref_axis',(1.,0.,0.));
#15491=DIRECTION('center_axis',(0.,1.,0.));
#15492=DIRECTION('ref_axis',(0.429672959082026,0.,-0.902984578070797));
#15493=DIRECTION('center_axis',(0.,-1.,0.));
#15494=DIRECTION('ref_axis',(1.,0.,0.));
#15495=DIRECTION('center_axis',(0.,-1.,0.));
#15496=DIRECTION('ref_axis',(1.,0.,0.));
#15497=DIRECTION('center_axis',(0.,-1.,0.));
#15498=DIRECTION('ref_axis',(1.,0.,0.));
#15499=DIRECTION('',(0.,-1.,0.));
#15500=DIRECTION('center_axis',(0.,1.,0.));
#15501=DIRECTION('ref_axis',(1.,0.,0.));
#15502=DIRECTION('center_axis',(0.,-1.,0.));
#15503=DIRECTION('ref_axis',(1.,0.,0.));
#15504=DIRECTION('',(0.,-1.,0.));
#15505=DIRECTION('center_axis',(0.,1.,0.));
#15506=DIRECTION('ref_axis',(1.,0.,0.));
#15507=DIRECTION('center_axis',(0.,-1.,0.));
#15508=DIRECTION('ref_axis',(1.,0.,0.));
#15509=DIRECTION('',(0.,-1.,0.));
#15510=DIRECTION('center_axis',(0.,1.,0.));
#15511=DIRECTION('ref_axis',(1.,0.,0.));
#15512=DIRECTION('center_axis',(0.,-1.,0.));
#15513=DIRECTION('ref_axis',(1.,0.,0.));
#15514=DIRECTION('',(0.,-1.,0.));
#15515=DIRECTION('center_axis',(0.,1.,0.));
#15516=DIRECTION('ref_axis',(1.,0.,0.));
#15517=DIRECTION('center_axis',(0.,-1.,0.));
#15518=DIRECTION('ref_axis',(1.,0.,0.));
#15519=DIRECTION('',(0.,-1.,0.));
#15520=DIRECTION('center_axis',(0.,1.,0.));
#15521=DIRECTION('ref_axis',(1.,0.,0.));
#15522=DIRECTION('center_axis',(0.,-1.,0.));
#15523=DIRECTION('ref_axis',(1.,0.,0.));
#15524=DIRECTION('',(0.,-1.,0.));
#15525=DIRECTION('center_axis',(0.,1.,0.));
#15526=DIRECTION('ref_axis',(1.,0.,0.));
#15527=DIRECTION('center_axis',(0.,-1.,0.));
#15528=DIRECTION('ref_axis',(1.,0.,0.));
#15529=DIRECTION('',(0.,-1.,0.));
#15530=DIRECTION('center_axis',(0.,1.,0.));
#15531=DIRECTION('ref_axis',(1.,0.,0.));
#15532=DIRECTION('center_axis',(0.,-1.,0.));
#15533=DIRECTION('ref_axis',(1.,0.,0.));
#15534=DIRECTION('',(0.,-1.,0.));
#15535=DIRECTION('center_axis',(0.,1.,0.));
#15536=DIRECTION('ref_axis',(1.,0.,0.));
#15537=DIRECTION('center_axis',(0.,1.,0.));
#15538=DIRECTION('ref_axis',(1.,0.,0.));
#15539=DIRECTION('center_axis',(0.,-1.,0.));
#15540=DIRECTION('ref_axis',(1.,0.,0.));
#15541=DIRECTION('',(-0.707106781186539,0.707106781186556,8.65956056235484E-17));
#15542=DIRECTION('center_axis',(0.,-1.,0.));
#15543=DIRECTION('ref_axis',(1.,0.,0.));
#15544=DIRECTION('',(0.,-1.,0.));
#15545=DIRECTION('center_axis',(0.,-1.,0.));
#15546=DIRECTION('ref_axis',(1.,0.,0.));
#15547=DIRECTION('center_axis',(0.,1.,0.));
#15548=DIRECTION('ref_axis',(1.,0.,0.));
#15549=DIRECTION('center_axis',(0.,-1.,0.));
#15550=DIRECTION('ref_axis',(1.,0.,0.));
#15551=DIRECTION('',(-0.707106781186547,0.707106781186548,8.65956056235493E-17));
#15552=DIRECTION('center_axis',(0.,-1.,0.));
#15553=DIRECTION('ref_axis',(1.,0.,0.));
#15554=DIRECTION('',(0.,-1.,0.));
#15555=DIRECTION('center_axis',(0.,-1.,0.));
#15556=DIRECTION('ref_axis',(1.,0.,0.));
#15557=DIRECTION('center_axis',(0.,-1.,0.));
#15558=DIRECTION('ref_axis',(1.,0.,0.));
#15559=DIRECTION('',(0.,-1.,0.));
#15560=DIRECTION('center_axis',(0.,-1.,0.));
#15561=DIRECTION('ref_axis',(1.,0.,0.));
#15562=DIRECTION('center_axis',(0.,-1.,0.));
#15563=DIRECTION('ref_axis',(1.,0.,0.));
#15564=DIRECTION('',(0.,-1.,0.));
#15565=DIRECTION('center_axis',(0.,-1.,0.));
#15566=DIRECTION('ref_axis',(1.,0.,0.));
#15567=DIRECTION('center_axis',(0.,-1.,0.));
#15568=DIRECTION('ref_axis',(1.,0.,0.));
#15569=DIRECTION('',(0.,-1.,0.));
#15570=DIRECTION('center_axis',(0.,-1.,0.));
#15571=DIRECTION('ref_axis',(1.,0.,0.));
#15572=DIRECTION('center_axis',(0.,-1.,0.));
#15573=DIRECTION('ref_axis',(1.,0.,0.));
#15574=DIRECTION('',(0.,-1.,0.));
#15575=DIRECTION('center_axis',(0.,-1.,0.));
#15576=DIRECTION('ref_axis',(1.,0.,0.));
#15577=DIRECTION('center_axis',(0.,1.,0.));
#15578=DIRECTION('ref_axis',(1.,0.,0.));
#15579=DIRECTION('center_axis',(0.,-1.,0.));
#15580=DIRECTION('ref_axis',(1.,0.,0.));
#15581=DIRECTION('',(-0.707106781186547,0.707106781186548,8.65956056235493E-17));
#15582=DIRECTION('center_axis',(0.,-1.,0.));
#15583=DIRECTION('ref_axis',(1.,0.,0.));
#15584=DIRECTION('',(0.,-1.,0.));
#15585=DIRECTION('center_axis',(0.,-1.,0.));
#15586=DIRECTION('ref_axis',(1.,0.,0.));
#15587=DIRECTION('center_axis',(0.,1.,0.));
#15588=DIRECTION('ref_axis',(1.,0.,0.));
#15589=DIRECTION('center_axis',(0.,-1.,0.));
#15590=DIRECTION('ref_axis',(1.,0.,0.));
#15591=DIRECTION('',(-0.707106781186539,0.707106781186556,8.65956056235484E-17));
#15592=DIRECTION('center_axis',(0.,-1.,0.));
#15593=DIRECTION('ref_axis',(1.,0.,0.));
#15594=DIRECTION('',(0.,-1.,0.));
#15595=DIRECTION('center_axis',(0.,-1.,0.));
#15596=DIRECTION('ref_axis',(1.,0.,0.));
#15597=DIRECTION('center_axis',(0.,1.,0.));
#15598=DIRECTION('ref_axis',(1.,0.,0.));
#15599=DIRECTION('',(-0.85716730070211,0.515038074910058,1.04972719113862E-16));
#15600=DIRECTION('center_axis',(0.,1.,0.));
#15601=DIRECTION('ref_axis',(1.,0.,0.));
#15602=DIRECTION('',(-0.85716730070211,0.515038074910058,1.04972719113862E-16));
#15603=DIRECTION('center_axis',(0.,1.,0.));
#15604=DIRECTION('ref_axis',(1.,0.,0.));
#15605=DIRECTION('',(-0.85716730070211,0.515038074910058,1.04972719113862E-16));
#15606=DIRECTION('center_axis',(0.,1.,0.));
#15607=DIRECTION('ref_axis',(1.,0.,0.));
#15608=DIRECTION('',(-0.85716730070211,0.515038074910058,1.04972719113862E-16));
#15609=DIRECTION('center_axis',(0.,1.,0.));
#15610=DIRECTION('ref_axis',(1.,0.,0.));
#15611=DIRECTION('',(-0.85716730070211,0.515038074910058,1.04972719113862E-16));
#15612=DIRECTION('center_axis',(0.,1.,0.));
#15613=DIRECTION('ref_axis',(1.,0.,0.));
#15614=DIRECTION('',(-0.85716730070211,0.515038074910058,1.04972719113862E-16));
#15615=DIRECTION('center_axis',(0.,1.,0.));
#15616=DIRECTION('ref_axis',(1.,0.,0.));
#15617=DIRECTION('',(-0.85716730070211,0.515038074910058,1.04972719113862E-16));
#15618=DIRECTION('center_axis',(0.,1.,0.));
#15619=DIRECTION('ref_axis',(1.,0.,0.));
#15620=DIRECTION('',(-0.85716730070211,0.515038074910058,1.04972719113862E-16));
#15621=DIRECTION('center_axis',(0.707106781186548,0.707106781186548,0.));
#15622=DIRECTION('ref_axis',(0.,0.,-1.));
#15623=DIRECTION('',(0.577350269189626,-0.577350269189626,0.577350269189626));
#15624=DIRECTION('',(0.,0.,-1.));
#15625=DIRECTION('',(0.577350269189626,-0.577350269189626,-0.577350269189626));
#15626=DIRECTION('center_axis',(0.,0.707106781186548,0.707106781186548));
#15627=DIRECTION('ref_axis',(1.,0.,0.));
#15628=DIRECTION('',(-0.577350269189626,-0.577350269189626,0.577350269189626));
#15629=DIRECTION('',(1.,0.,0.));
#15630=DIRECTION('center_axis',(-0.707106781186548,0.707106781186548,0.));
#15631=DIRECTION('ref_axis',(0.,0.,1.));
#15632=DIRECTION('',(-0.577350269189626,-0.577350269189626,-0.577350269189626));
#15633=DIRECTION('',(0.,0.,1.));
#15634=DIRECTION('center_axis',(0.,0.707106781186548,-0.707106781186548));
#15635=DIRECTION('ref_axis',(-1.,0.,0.));
#15636=DIRECTION('',(-1.,0.,0.));
#15637=DIRECTION('center_axis',(0.,0.,-1.));
#15638=DIRECTION('ref_axis',(-1.,0.,0.));
#15639=DIRECTION('',(0.,1.,0.));
#15640=DIRECTION('',(1.,0.,0.));
#15641=DIRECTION('',(0.,1.,0.));
#15642=DIRECTION('center_axis',(1.,0.,0.));
#15643=DIRECTION('ref_axis',(0.,0.,-1.));
#15644=DIRECTION('',(0.,1.,0.));
#15645=DIRECTION('',(0.,0.,1.));
#15646=DIRECTION('center_axis',(-1.,0.,0.));
#15647=DIRECTION('ref_axis',(0.,0.,1.));
#15648=DIRECTION('',(0.,0.,-1.));
#15649=DIRECTION('',(0.,1.,0.));
#15650=DIRECTION('center_axis',(0.,0.,1.));
#15651=DIRECTION('ref_axis',(1.,0.,0.));
#15652=DIRECTION('',(-1.,0.,0.));
#15653=DIRECTION('center_axis',(0.,1.,0.));
#15654=DIRECTION('ref_axis',(1.,0.,0.));
#19002=CARTESIAN_POINT('',(0.,0.,0.));
#19003=CARTESIAN_POINT('Origin',(137.6,52.2248,48.));
#19004=CARTESIAN_POINT('',(138.782171994385,52.0748000118745,43.917724971177));
#19005=CARTESIAN_POINT('',(137.907849128401,52.3748,43.4604263510609));
#19006=CARTESIAN_POINT('Ctrl Pts',(138.782171998071,52.0748000121059,43.9177249639598));
#19007=CARTESIAN_POINT('Ctrl Pts',(138.651976643645,52.1016376463417,43.8520818493382));
#19008=CARTESIAN_POINT('Ctrl Pts',(138.526269777382,52.1358607961625,43.7875586696316));
#19009=CARTESIAN_POINT('Ctrl Pts',(138.232505475659,52.2319385954063,43.6345597499497));
#19010=CARTESIAN_POINT('Ctrl Pts',(138.06786919821,52.2992964813024,43.5469549723518));
#19011=CARTESIAN_POINT('Ctrl Pts',(137.907849128401,52.3748000000001,43.4604263510608));
#19012=CARTESIAN_POINT('',(140.928421084005,52.3748,44.8977245306789));
#19013=CARTESIAN_POINT('Origin',(137.6,52.3748,48.));
#19014=CARTESIAN_POINT('',(140.022078380249,52.0748000118746,44.5077176008821));
#19015=CARTESIAN_POINT('Ctrl Pts',(140.928421084005,52.3748,44.897724530679));
#19016=CARTESIAN_POINT('Ctrl Pts',(140.760391286209,52.2993184802566,44.828152047826));
#19017=CARTESIAN_POINT('Ctrl Pts',(140.588616367553,52.2319776911148,44.755677770846));
#19018=CARTESIAN_POINT('Ctrl Pts',(140.284602785751,52.1358885558017,44.6242337550021));
#19019=CARTESIAN_POINT('Ctrl Pts',(140.155192346908,52.1016485689512,44.5673651425763));
#19020=CARTESIAN_POINT('Ctrl Pts',(140.022078383524,52.074800012106,44.5077175934691));
#19021=CARTESIAN_POINT('Origin',(137.6,52.0748,48.));
#19022=CARTESIAN_POINT('Origin',(90.,52.3748,0.));
#19023=CARTESIAN_POINT('',(146.35,52.3748,-56.35));
#19024=CARTESIAN_POINT('',(146.35,52.3748,56.35));
#19025=CARTESIAN_POINT('',(146.35,52.3748,28.575));
#19026=CARTESIAN_POINT('',(33.65,52.3748,-56.35));
#19027=CARTESIAN_POINT('',(118.575,52.3748,-56.35));
#19028=CARTESIAN_POINT('',(33.65,52.3748,56.35));
#19029=CARTESIAN_POINT('',(33.65,52.3748,-28.575));
#19030=CARTESIAN_POINT('',(61.425,52.3748,56.35));
#19031=CARTESIAN_POINT('',(114.05,52.3748,48.));
#19032=CARTESIAN_POINT('Origin',(118.6,52.3748,48.));
#19033=CARTESIAN_POINT('',(56.85,52.3748,-48.));
#19034=CARTESIAN_POINT('Origin',(61.4,52.3748,-48.));
#19035=CARTESIAN_POINT('',(56.85,52.3748,48.));
#19036=CARTESIAN_POINT('Origin',(61.4,52.3748,48.));
#19037=CARTESIAN_POINT('',(60.975,52.3748,19.05));
#19038=CARTESIAN_POINT('Origin',(64.6,52.3748,19.05));
#19039=CARTESIAN_POINT('',(140.928421084005,52.3748,-44.8977245306789));
#19040=CARTESIAN_POINT('',(137.907849128401,52.3748,-43.4604263510609));
#19041=CARTESIAN_POINT('Origin',(137.6,52.3748,-48.));
#19042=CARTESIAN_POINT('Origin',(140.8,52.3748,-41.275));
#19043=CARTESIAN_POINT('Origin',(140.8,52.3748,41.275));
#19044=CARTESIAN_POINT('',(111.775,52.3748,-19.05));
#19045=CARTESIAN_POINT('Origin',(115.4,52.3748,-19.05));
#19046=CARTESIAN_POINT('',(60.975,52.3748,-19.05));
#19047=CARTESIAN_POINT('Origin',(64.6,52.3748,-19.05));
#19048=CARTESIAN_POINT('',(39.071578915995,52.3748,44.8977245306789));
#19049=CARTESIAN_POINT('',(42.0921508715986,52.3748,43.4604263510609));
#19050=CARTESIAN_POINT('Origin',(42.4,52.3748,48.));
#19051=CARTESIAN_POINT('Origin',(39.2,52.3748,41.275));
#19052=CARTESIAN_POINT('',(42.0921508715986,52.3748,-43.4604263510609));
#19053=CARTESIAN_POINT('',(39.071578915995,52.3748,-44.8977245306789));
#19054=CARTESIAN_POINT('Origin',(42.4,52.3748,-48.));
#19055=CARTESIAN_POINT('Origin',(39.2,52.3748,-41.275));
#19056=CARTESIAN_POINT('',(111.775,52.3748,19.05));
#19057=CARTESIAN_POINT('Origin',(115.4,52.3748,19.05));
#19058=CARTESIAN_POINT('',(114.05,52.3748,-48.));
#19059=CARTESIAN_POINT('Origin',(118.6,52.3748,-48.));
#19060=CARTESIAN_POINT('Origin',(118.6,52.2248,48.));
#19061=CARTESIAN_POINT('',(114.35,52.0748,48.));
#19062=CARTESIAN_POINT('Origin',(118.6,52.0748,48.));
#19063=CARTESIAN_POINT('',(114.2,52.2248,48.));
#19064=CARTESIAN_POINT('Origin',(118.6,52.3748,48.));
#19065=CARTESIAN_POINT('',(114.35,47.1748,48.));
#19066=CARTESIAN_POINT('',(114.35,52.3748,48.));
#19067=CARTESIAN_POINT('Origin',(118.6,47.1748,48.));
#19068=CARTESIAN_POINT('Origin',(42.4,52.2248,-48.));
#19069=CARTESIAN_POINT('',(41.2178280056156,52.0748000118745,-43.917724971177));
#19070=CARTESIAN_POINT('Ctrl Pts',(41.217828001929,52.074800012106,-43.9177249639597));
#19071=CARTESIAN_POINT('Ctrl Pts',(41.3480233563548,52.1016376463417,-43.8520818493381));
#19072=CARTESIAN_POINT('Ctrl Pts',(41.4737302226176,52.1358607961625,-43.7875586696315));
#19073=CARTESIAN_POINT('Ctrl Pts',(41.7674945243411,52.2319385954063,-43.6345597499497));
#19074=CARTESIAN_POINT('Ctrl Pts',(41.9321308017903,52.2992964813023,-43.5469549723519));
#19075=CARTESIAN_POINT('Ctrl Pts',(42.0921508715986,52.3748,-43.4604263510609));
#19076=CARTESIAN_POINT('',(39.9779216197509,52.0748000118745,-44.5077176008821));
#19077=CARTESIAN_POINT('Ctrl Pts',(39.071578915995,52.3748,-44.897724530679));
#19078=CARTESIAN_POINT('Ctrl Pts',(39.2396087137915,52.2993184802566,-44.828152047826));
#19079=CARTESIAN_POINT('Ctrl Pts',(39.4113836324468,52.2319776911147,-44.755677770846));
#19080=CARTESIAN_POINT('Ctrl Pts',(39.7153972142493,52.1358885558017,-44.6242337550021));
#19081=CARTESIAN_POINT('Ctrl Pts',(39.8448076530922,52.1016485689511,-44.5673651425763));
#19082=CARTESIAN_POINT('Ctrl Pts',(39.9779216164758,52.074800012106,-44.5077175934691));
#19083=CARTESIAN_POINT('Origin',(42.4,52.0748,-48.));
#19084=CARTESIAN_POINT('Origin',(61.4,52.2248,-48.));
#19085=CARTESIAN_POINT('',(57.15,52.0748,-48.));
#19086=CARTESIAN_POINT('Origin',(61.4,52.0748,-48.));
#19087=CARTESIAN_POINT('',(57.,52.2248,-48.));
#19088=CARTESIAN_POINT('Origin',(61.4,52.3748,-48.));
#19089=CARTESIAN_POINT('',(57.15,47.1748,-48.));
#19090=CARTESIAN_POINT('',(57.15,52.3748,-48.));
#19091=CARTESIAN_POINT('Origin',(61.4,47.1748,-48.));
#19092=CARTESIAN_POINT('Origin',(42.4,52.2248,48.));
#19093=CARTESIAN_POINT('',(39.9779216197508,52.0748000118745,44.5077176008821));
#19094=CARTESIAN_POINT('Ctrl Pts',(39.9779216164758,52.074800012106,44.5077175934691));
#19095=CARTESIAN_POINT('Ctrl Pts',(39.8448618069091,52.1016376463417,44.5673408765836));
#19096=CARTESIAN_POINT('Ctrl Pts',(39.7155022091841,52.1358607961625,44.6241876128267));
#19097=CARTESIAN_POINT('Ctrl Pts',(39.4114832568764,52.2319385954063,44.7556357433902));
#19098=CARTESIAN_POINT('Ctrl Pts',(39.2396576857764,52.2992964813023,44.82813177105));
#19099=CARTESIAN_POINT('Ctrl Pts',(39.071578915995,52.3748,44.897724530679));
#19100=CARTESIAN_POINT('',(41.2178280056156,52.0748000118745,43.917724971177));
#19101=CARTESIAN_POINT('Ctrl Pts',(42.0921508715986,52.3748,43.4604263510609));
#19102=CARTESIAN_POINT('Ctrl Pts',(41.9321774257658,52.2993184802566,43.5469297610873));
#19103=CARTESIAN_POINT('Ctrl Pts',(41.7675899759767,52.2319776911147,43.6345089531068));
#19104=CARTESIAN_POINT('Ctrl Pts',(41.4738322546896,52.1358885558017,43.7875063008149));
#19105=CARTESIAN_POINT('Ctrl Pts',(41.3480763443713,52.1016485689512,43.8520551333431));
#19106=CARTESIAN_POINT('Ctrl Pts',(41.217828001929,52.074800012106,43.9177249639597));
#19107=CARTESIAN_POINT('Origin',(42.4,52.0748,48.));
#19108=CARTESIAN_POINT('Origin',(61.4,52.2248,48.));
#19109=CARTESIAN_POINT('',(57.15,52.0748,48.));
#19110=CARTESIAN_POINT('Origin',(61.4,52.0748,48.));
#19111=CARTESIAN_POINT('',(57.,52.2248,48.));
#19112=CARTESIAN_POINT('Origin',(61.4,52.3748,48.));
#19113=CARTESIAN_POINT('',(57.15,47.1748,48.));
#19114=CARTESIAN_POINT('',(57.15,52.3748,48.));
#19115=CARTESIAN_POINT('Origin',(61.4,47.1748,48.));
#19116=CARTESIAN_POINT('Origin',(118.6,52.2248,-48.));
#19117=CARTESIAN_POINT('',(114.35,52.0748,-48.));
#19118=CARTESIAN_POINT('Origin',(118.6,52.0748,-48.));
#19119=CARTESIAN_POINT('',(114.2,52.2248,-48.));
#19120=CARTESIAN_POINT('Origin',(118.6,52.3748,-48.));
#19121=CARTESIAN_POINT('',(114.35,47.1748,-48.));
#19122=CARTESIAN_POINT('',(114.35,52.3748,-48.));
#19123=CARTESIAN_POINT('Origin',(118.6,47.1748,-48.));
#19124=CARTESIAN_POINT('Origin',(137.6,52.2248,-48.));
#19125=CARTESIAN_POINT('',(140.022078380249,52.0748000118745,-44.5077176008821));
#19126=CARTESIAN_POINT('Ctrl Pts',(140.022078383524,52.074800012106,-44.5077175934691));
#19127=CARTESIAN_POINT('Ctrl Pts',(140.155138193091,52.1016376463417,-44.5673408765836));
#19128=CARTESIAN_POINT('Ctrl Pts',(140.284497790816,52.1358607961625,-44.6241876128266));
#19129=CARTESIAN_POINT('Ctrl Pts',(140.588516743124,52.2319385954063,-44.7556357433902));
#19130=CARTESIAN_POINT('Ctrl Pts',(140.760342314224,52.2992964813023,-44.8281317710499));
#19131=CARTESIAN_POINT('Ctrl Pts',(140.928421084005,52.3748,-44.8977245306789));
#19132=CARTESIAN_POINT('',(138.782171994385,52.0748000118745,-43.917724971177));
#19133=CARTESIAN_POINT('Ctrl Pts',(137.907849128401,52.3748000000001,-43.4604263510607));
#19134=CARTESIAN_POINT('Ctrl Pts',(138.067822574234,52.2993184802567,-43.5469297610872));
#19135=CARTESIAN_POINT('Ctrl Pts',(138.232410024023,52.2319776911148,-43.6345089531068));
#19136=CARTESIAN_POINT('Ctrl Pts',(138.526167745311,52.1358885558016,-43.7875063008149));
#19137=CARTESIAN_POINT('Ctrl Pts',(138.651923655629,52.1016485689511,-43.8520551333431));
#19138=CARTESIAN_POINT('Ctrl Pts',(138.782171998071,52.0748000121059,-43.9177249639598));
#19139=CARTESIAN_POINT('Origin',(137.6,52.0748,-48.));
#19140=CARTESIAN_POINT('Origin',(137.6,52.3748,-48.));
#19141=CARTESIAN_POINT('',(139.13467476064,51.9748,-44.0367597374051));
#19142=CARTESIAN_POINT('Ctrl Pts',(139.13467476064,51.9748000000001,-44.036759737405));
#19143=CARTESIAN_POINT('Ctrl Pts',(139.018142335558,51.9963321756324,-43.9916352030039));
#19144=CARTESIAN_POINT('Ctrl Pts',(138.899881099053,52.0304589029105,-43.9518119506536));
#19145=CARTESIAN_POINT('Ctrl Pts',(138.782171996941,52.0748000225489,-43.9177249762358));
#19146=CARTESIAN_POINT('',(139.13467476064,47.1748,-44.0367597374051));
#19147=CARTESIAN_POINT('',(139.13467476064,52.3748,-44.0367597374051));
#19148=CARTESIAN_POINT('',(139.707364790884,47.1748,-44.3092665175952));
#19149=CARTESIAN_POINT('Origin',(137.6,47.1748,-48.));
#19150=CARTESIAN_POINT('',(139.707364790884,51.9748,-44.3092665175952));
#19151=CARTESIAN_POINT('',(139.707364790884,52.3748,-44.3092665175952));
#19152=CARTESIAN_POINT('Ctrl Pts',(140.022078374711,52.074800022549,-44.5077176020895));
#19153=CARTESIAN_POINT('Ctrl Pts',(139.921436670535,52.0304833142233,-44.4379173776217));
#19154=CARTESIAN_POINT('Ctrl Pts',(139.81593061941,51.9963413043493,-44.3712563105783));
#19155=CARTESIAN_POINT('Ctrl Pts',(139.707364790884,51.9748000000001,-44.3092665175953));
#19156=CARTESIAN_POINT('Origin',(137.6,47.1748,-48.));
#19157=CARTESIAN_POINT('Origin',(140.8,47.1748,-41.275));
#19158=CARTESIAN_POINT('',(135.,47.1748,-48.));
#19159=CARTESIAN_POINT('Origin',(137.6,47.1748,-48.));
#19160=CARTESIAN_POINT('Origin',(118.6,47.1748,-48.));
#19161=CARTESIAN_POINT('',(116.,47.1748,-48.));
#19162=CARTESIAN_POINT('Origin',(118.6,47.1748,-48.));
#19163=CARTESIAN_POINT('Origin',(61.4,47.1748,48.));
#19164=CARTESIAN_POINT('',(58.8,47.1748,48.));
#19165=CARTESIAN_POINT('Origin',(61.4,47.1748,48.));
#19166=CARTESIAN_POINT('Origin',(42.4,52.3748,48.));
#19167=CARTESIAN_POINT('',(40.8653252393596,51.9748,44.0367597374051));
#19168=CARTESIAN_POINT('Ctrl Pts',(40.8653252393596,51.9748,44.0367597374051));
#19169=CARTESIAN_POINT('Ctrl Pts',(40.9818576644415,51.9963321756324,43.991635203004));
#19170=CARTESIAN_POINT('Ctrl Pts',(41.1001189009476,52.0304589029105,43.9518119506536));
#19171=CARTESIAN_POINT('Ctrl Pts',(41.2178280030595,52.074800022549,43.9177249762357));
#19172=CARTESIAN_POINT('',(40.8653252393596,47.1748,44.0367597374051));
#19173=CARTESIAN_POINT('',(40.8653252393596,52.3748,44.0367597374051));
#19174=CARTESIAN_POINT('',(40.2926352091164,47.1748,44.3092665175952));
#19175=CARTESIAN_POINT('Origin',(42.4,47.1748,48.));
#19176=CARTESIAN_POINT('',(40.2926352091163,51.9748,44.3092665175952));
#19177=CARTESIAN_POINT('',(40.2926352091164,52.3748,44.3092665175952));
#19178=CARTESIAN_POINT('Ctrl Pts',(39.9779216252887,52.074800022549,44.5077176020895));
#19179=CARTESIAN_POINT('Ctrl Pts',(40.0785633294647,52.0304833142233,44.4379173776217));
#19180=CARTESIAN_POINT('Ctrl Pts',(40.1840693805898,51.9963413043492,44.3712563105783));
#19181=CARTESIAN_POINT('Ctrl Pts',(40.2926352091163,51.9748,44.3092665175952));
#19182=CARTESIAN_POINT('Origin',(42.4,47.1748,48.));
#19183=CARTESIAN_POINT('Origin',(39.2,47.1748,41.275));
#19184=CARTESIAN_POINT('',(39.8,47.1748,48.));
#19185=CARTESIAN_POINT('Origin',(42.4,47.1748,48.));
#19186=CARTESIAN_POINT('Origin',(61.4,47.1748,-48.));
#19187=CARTESIAN_POINT('',(58.8,47.1748,-48.));
#19188=CARTESIAN_POINT('Origin',(61.4,47.1748,-48.));
#19189=CARTESIAN_POINT('Origin',(42.4,52.3748,-48.));
#19190=CARTESIAN_POINT('',(40.2926352091163,51.9748,-44.3092665175952));
#19191=CARTESIAN_POINT('Ctrl Pts',(40.2926352091163,51.9748,-44.3092665175952));
#19192=CARTESIAN_POINT('Ctrl Pts',(40.1841153883286,51.9963321756324,-44.3712300407083));
#19193=CARTESIAN_POINT('Ctrl Pts',(40.0786187667076,52.0304589029105,-44.437878929028));
#19194=CARTESIAN_POINT('Ctrl Pts',(39.9779216252887,52.074800022549,-44.5077176020895));
#19195=CARTESIAN_POINT('',(40.2926352091164,47.1748,-44.3092665175952));
#19196=CARTESIAN_POINT('',(40.2926352091164,52.3748,-44.3092665175952));
#19197=CARTESIAN_POINT('',(40.8653252393596,47.1748,-44.0367597374051));
#19198=CARTESIAN_POINT('Origin',(42.4,47.1748,-48.));
#19199=CARTESIAN_POINT('',(40.8653252393596,51.9748,-44.0367597374051));
#19200=CARTESIAN_POINT('',(40.8653252393596,52.3748,-44.0367597374051));
#19201=CARTESIAN_POINT('Ctrl Pts',(41.2178280030594,52.074800022549,-43.9177249762357));
#19202=CARTESIAN_POINT('Ctrl Pts',(41.1001837038604,52.0304833142233,-43.9517931846007));
#19203=CARTESIAN_POINT('Ctrl Pts',(40.98190706918,51.9963413043492,-43.9916160721413));
#19204=CARTESIAN_POINT('Ctrl Pts',(40.8653252393596,51.9748,-44.0367597374051));
#19205=CARTESIAN_POINT('Origin',(42.4,47.1748,-48.));
#19206=CARTESIAN_POINT('Origin',(39.2,47.1748,-41.275));
#19207=CARTESIAN_POINT('',(39.8,47.1748,-48.));
#19208=CARTESIAN_POINT('Origin',(42.4,47.1748,-48.));
#19209=CARTESIAN_POINT('Origin',(118.6,47.1748,48.));
#19210=CARTESIAN_POINT('',(116.,47.1748,48.));
#19211=CARTESIAN_POINT('Origin',(118.6,47.1748,48.));
#19212=CARTESIAN_POINT('Origin',(137.6,52.3748,48.));
#19213=CARTESIAN_POINT('',(139.707364790884,51.9748,44.3092665175952));
#19214=CARTESIAN_POINT('Ctrl Pts',(139.707364790884,51.9748000000001,44.3092665175953));
#19215=CARTESIAN_POINT('Ctrl Pts',(139.815884611672,51.9963321756325,44.3712300407084));
#19216=CARTESIAN_POINT('Ctrl Pts',(139.921381233292,52.0304589029105,44.4378789290281));
#19217=CARTESIAN_POINT('Ctrl Pts',(140.022078374711,52.074800022549,44.5077176020895));
#19218=CARTESIAN_POINT('',(139.707364790884,47.1748,44.3092665175952));
#19219=CARTESIAN_POINT('',(139.707364790884,52.3748,44.3092665175952));
#19220=CARTESIAN_POINT('',(139.13467476064,47.1748,44.0367597374051));
#19221=CARTESIAN_POINT('Origin',(137.6,47.1748,48.));
#19222=CARTESIAN_POINT('',(139.13467476064,51.9748,44.0367597374051));
#19223=CARTESIAN_POINT('',(139.13467476064,52.3748,44.0367597374051));
#19224=CARTESIAN_POINT('Ctrl Pts',(138.782171996941,52.074800022549,43.9177249762358));
#19225=CARTESIAN_POINT('Ctrl Pts',(138.89981629614,52.0304833142233,43.9517931846007));
#19226=CARTESIAN_POINT('Ctrl Pts',(139.01809293082,51.9963413043493,43.9916160721412));
#19227=CARTESIAN_POINT('Ctrl Pts',(139.13467476064,51.9748000000001,44.036759737405));
#19228=CARTESIAN_POINT('Origin',(137.6,47.1748,48.));
#19229=CARTESIAN_POINT('Origin',(140.8,47.1748,41.275));
#19230=CARTESIAN_POINT('',(135.,47.1748,48.));
#19231=CARTESIAN_POINT('Origin',(137.6,47.1748,48.));
#19232=CARTESIAN_POINT('Origin',(140.8,52.1748,-41.275));
#19233=CARTESIAN_POINT('',(137.575,51.9748,-41.275));
#19234=CARTESIAN_POINT('Origin',(140.8,51.9748,-41.275));
#19235=CARTESIAN_POINT('Origin',(140.8,51.9748,-41.275));
#19236=CARTESIAN_POINT('Origin',(39.2,52.1748,41.275));
#19237=CARTESIAN_POINT('',(35.975,51.9748,41.275));
#19238=CARTESIAN_POINT('Origin',(39.2,51.9748,41.275));
#19239=CARTESIAN_POINT('Origin',(39.2,51.9748,41.275));
#19240=CARTESIAN_POINT('Origin',(39.2,52.1748,-41.275));
#19241=CARTESIAN_POINT('',(35.975,51.9748,-41.275));
#19242=CARTESIAN_POINT('Origin',(39.2,51.9748,-41.275));
#19243=CARTESIAN_POINT('Origin',(39.2,51.9748,-41.275));
#19244=CARTESIAN_POINT('Origin',(140.8,52.1748,41.275));
#19245=CARTESIAN_POINT('',(137.575,51.9748,41.275));
#19246=CARTESIAN_POINT('Origin',(140.8,51.9748,41.275));
#19247=CARTESIAN_POINT('Origin',(140.8,51.9748,41.275));
#19248=CARTESIAN_POINT('Origin',(137.6,52.3748,-48.));
#19249=CARTESIAN_POINT('',(135.,39.6748,-48.));
#19250=CARTESIAN_POINT('',(135.,52.3748,-48.));
#19251=CARTESIAN_POINT('Origin',(137.6,39.6748,-48.));
#19252=CARTESIAN_POINT('Origin',(118.6,52.3748,-48.));
#19253=CARTESIAN_POINT('',(116.,39.6748,-48.));
#19254=CARTESIAN_POINT('',(116.,52.3748,-48.));
#19255=CARTESIAN_POINT('Origin',(118.6,39.6748,-48.));
#19256=CARTESIAN_POINT('Origin',(61.4,52.3748,48.));
#19257=CARTESIAN_POINT('',(58.8,39.6748,48.));
#19258=CARTESIAN_POINT('',(58.8,52.3748,48.));
#19259=CARTESIAN_POINT('Origin',(61.4,39.6748,48.));
#19260=CARTESIAN_POINT('Origin',(42.4,52.3748,48.));
#19261=CARTESIAN_POINT('',(39.8,39.6748,48.));
#19262=CARTESIAN_POINT('',(39.8,52.3748,48.));
#19263=CARTESIAN_POINT('Origin',(42.4,39.6748,48.));
#19264=CARTESIAN_POINT('Origin',(61.4,52.3748,-48.));
#19265=CARTESIAN_POINT('',(58.8,39.6748,-48.));
#19266=CARTESIAN_POINT('',(58.8,52.3748,-48.));
#19267=CARTESIAN_POINT('Origin',(61.4,39.6748,-48.));
#19268=CARTESIAN_POINT('Origin',(42.4,52.3748,-48.));
#19269=CARTESIAN_POINT('',(39.8,39.6748,-48.));
#19270=CARTESIAN_POINT('',(39.8,52.3748,-48.));
#19271=CARTESIAN_POINT('Origin',(42.4,39.6748,-48.));
#19272=CARTESIAN_POINT('Origin',(118.6,52.3748,48.));
#19273=CARTESIAN_POINT('',(116.,39.6748,48.));
#19274=CARTESIAN_POINT('',(116.,52.3748,48.));
#19275=CARTESIAN_POINT('Origin',(118.6,39.6748,48.));
#19276=CARTESIAN_POINT('Origin',(137.6,52.3748,48.));
#19277=CARTESIAN_POINT('',(135.,39.6748,48.));
#19278=CARTESIAN_POINT('',(135.,52.3748,48.));
#19279=CARTESIAN_POINT('Origin',(137.6,39.6748,48.));
#19280=CARTESIAN_POINT('Origin',(115.4,52.1748,19.05));
#19281=CARTESIAN_POINT('',(112.175,51.9748,19.05));
#19282=CARTESIAN_POINT('Origin',(115.4,51.9748,19.05));
#19283=CARTESIAN_POINT('',(111.975,52.1748,19.05));
#19284=CARTESIAN_POINT('Origin',(115.4,52.3748,19.05));
#19285=CARTESIAN_POINT('',(112.175,42.3748,19.05));
#19286=CARTESIAN_POINT('',(112.175,52.3748,19.05));
#19287=CARTESIAN_POINT('Origin',(115.4,42.3748,19.05));
#19288=CARTESIAN_POINT('Origin',(64.6,52.1748,19.05));
#19289=CARTESIAN_POINT('',(61.375,51.9748,19.05));
#19290=CARTESIAN_POINT('Origin',(64.6,51.9748,19.05));
#19291=CARTESIAN_POINT('',(61.175,52.1748,19.05));
#19292=CARTESIAN_POINT('Origin',(64.6,52.3748,19.05));
#19293=CARTESIAN_POINT('',(61.375,42.3748,19.05));
#19294=CARTESIAN_POINT('',(61.375,52.3748,19.05));
#19295=CARTESIAN_POINT('Origin',(64.6,42.3748,19.05));
#19296=CARTESIAN_POINT('Origin',(39.2,52.3748,-41.275));
#19297=CARTESIAN_POINT('',(35.975,42.3748,-41.275));
#19298=CARTESIAN_POINT('',(35.975,52.3748,-41.275));
#19299=CARTESIAN_POINT('Origin',(39.2,42.3748,-41.275));
#19300=CARTESIAN_POINT('Origin',(140.8,52.3748,-41.275));
#19301=CARTESIAN_POINT('',(137.575,42.3748,-41.275));
#19302=CARTESIAN_POINT('',(137.575,52.3748,-41.275));
#19303=CARTESIAN_POINT('Origin',(140.8,42.3748,-41.275));
#19304=CARTESIAN_POINT('Origin',(39.2,52.3748,41.275));
#19305=CARTESIAN_POINT('',(35.975,42.3748,41.275));
#19306=CARTESIAN_POINT('',(35.975,52.3748,41.275));
#19307=CARTESIAN_POINT('Origin',(39.2,42.3748,41.275));
#19308=CARTESIAN_POINT('Origin',(140.8,52.3748,41.275));
#19309=CARTESIAN_POINT('',(137.575,42.3748,41.275));
#19310=CARTESIAN_POINT('',(137.575,52.3748,41.275));
#19311=CARTESIAN_POINT('Origin',(140.8,42.3748,41.275));
#19312=CARTESIAN_POINT('Origin',(64.6,52.1748,-19.05));
#19313=CARTESIAN_POINT('',(61.375,51.9748,-19.05));
#19314=CARTESIAN_POINT('Origin',(64.6,51.9748,-19.05));
#19315=CARTESIAN_POINT('',(61.175,52.1748,-19.05));
#19316=CARTESIAN_POINT('Origin',(64.6,52.3748,-19.05));
#19317=CARTESIAN_POINT('',(61.375,42.3748,-19.05));
#19318=CARTESIAN_POINT('',(61.375,52.3748,-19.05));
#19319=CARTESIAN_POINT('Origin',(64.6,42.3748,-19.05));
#19320=CARTESIAN_POINT('Origin',(115.4,52.1748,-19.05));
#19321=CARTESIAN_POINT('',(112.175,51.9748,-19.05));
#19322=CARTESIAN_POINT('Origin',(115.4,51.9748,-19.05));
#19323=CARTESIAN_POINT('',(111.975,52.1748,-19.05));
#19324=CARTESIAN_POINT('Origin',(115.4,52.3748,-19.05));
#19325=CARTESIAN_POINT('',(112.175,42.3748,-19.05));
#19326=CARTESIAN_POINT('',(112.175,52.3748,-19.05));
#19327=CARTESIAN_POINT('Origin',(115.4,42.3748,-19.05));
#19328=CARTESIAN_POINT('Origin',(115.4,42.3748,19.05));
#19329=CARTESIAN_POINT('',(115.4,40.4370245036361,19.05));
#19330=CARTESIAN_POINT('',(112.175,42.3748,19.05));
#19331=CARTESIAN_POINT('Origin',(115.4,42.3748,-19.05));
#19332=CARTESIAN_POINT('',(115.4,40.4370245036361,-19.05));
#19333=CARTESIAN_POINT('',(112.175,42.3748,-19.05));
#19334=CARTESIAN_POINT('Origin',(64.6,42.3748,19.05));
#19335=CARTESIAN_POINT('',(64.6,40.4370245036361,19.05));
#19336=CARTESIAN_POINT('',(61.375,42.3748,19.05));
#19337=CARTESIAN_POINT('Origin',(64.6,42.3748,-19.05));
#19338=CARTESIAN_POINT('',(64.6,40.4370245036361,-19.05));
#19339=CARTESIAN_POINT('',(61.375,42.3748,-19.05));
#19340=CARTESIAN_POINT('Origin',(140.8,42.3748,41.275));
#19341=CARTESIAN_POINT('',(140.8,40.4370245036361,41.275));
#19342=CARTESIAN_POINT('',(137.575,42.3748,41.275));
#19343=CARTESIAN_POINT('Origin',(140.8,42.3748,-41.275));
#19344=CARTESIAN_POINT('',(140.8,40.4370245036361,-41.275));
#19345=CARTESIAN_POINT('',(137.575,42.3748,-41.275));
#19346=CARTESIAN_POINT('Origin',(39.2,42.3748,41.275));
#19347=CARTESIAN_POINT('',(39.2,40.4370245036361,41.275));
#19348=CARTESIAN_POINT('',(35.975,42.3748,41.275));
#19349=CARTESIAN_POINT('Origin',(39.2,42.3748,-41.275));
#19350=CARTESIAN_POINT('',(39.2,40.4370245036361,-41.275));
#19351=CARTESIAN_POINT('',(35.975,42.3748,-41.275));
#19352=CARTESIAN_POINT('Origin',(146.75,51.9748,28.575));
#19353=CARTESIAN_POINT('',(147.15,51.5748,57.15));
#19354=CARTESIAN_POINT('',(146.35,52.3748,56.35));
#19355=CARTESIAN_POINT('',(147.15,51.5748,-57.15));
#19356=CARTESIAN_POINT('',(147.15,51.5748,28.575));
#19357=CARTESIAN_POINT('',(146.35,52.3748,-56.35));
#19358=CARTESIAN_POINT('Origin',(61.425,51.9748,56.75));
#19359=CARTESIAN_POINT('',(32.85,51.5748,57.15));
#19360=CARTESIAN_POINT('',(33.65,52.3748,56.35));
#19361=CARTESIAN_POINT('',(61.425,51.5748,57.15));
#19362=CARTESIAN_POINT('Origin',(33.25,51.9748,-28.575));
#19363=CARTESIAN_POINT('',(32.85,51.5748,-57.15));
#19364=CARTESIAN_POINT('',(33.65,52.3748,-56.35));
#19365=CARTESIAN_POINT('',(32.85,51.5748,-28.575));
#19366=CARTESIAN_POINT('Origin',(118.575,51.9748,-56.75));
#19367=CARTESIAN_POINT('',(118.575,51.5748,-57.15));
#19368=CARTESIAN_POINT('Origin',(147.15,39.6748,-57.15));
#19369=CARTESIAN_POINT('',(147.15,39.6748,-57.15));
#19370=CARTESIAN_POINT('',(147.15,39.6748,-57.15));
#19371=CARTESIAN_POINT('',(32.85,39.6748,-57.15));
#19372=CARTESIAN_POINT('',(32.85,39.6748,-57.15));
#19373=CARTESIAN_POINT('',(32.85,39.6748,-57.15));
#19374=CARTESIAN_POINT('Origin',(147.15,39.6748,57.15));
#19375=CARTESIAN_POINT('',(147.15,39.6748,57.15));
#19376=CARTESIAN_POINT('',(147.15,39.6748,57.15));
#19377=CARTESIAN_POINT('',(147.15,39.6748,-57.15));
#19378=CARTESIAN_POINT('Origin',(32.85,39.6748,-57.15));
#19379=CARTESIAN_POINT('',(32.85,39.6748,57.15));
#19380=CARTESIAN_POINT('',(32.85,39.6748,57.15));
#19381=CARTESIAN_POINT('',(32.85,39.6748,57.15));
#19382=CARTESIAN_POINT('Origin',(32.85,39.6748,57.15));
#19383=CARTESIAN_POINT('',(147.15,39.6748,57.15));
#19384=CARTESIAN_POINT('Origin',(90.,39.6748,0.));
#71774=UNCERTAINTY_MEASURE_WITH_UNIT(LENGTH_MEASURE(0.01),#71796,
'DISTANCE_ACCURACY_VALUE',
'Maximum model space distance between geometric entities at asserted c
onnectivities');
#71783=UNCERTAINTY_MEASURE_WITH_UNIT(LENGTH_MEASURE(0.01),#71796,
'DISTANCE_ACCURACY_VALUE',
'Maximum model space distance between geometric entities at asserted c
onnectivities');
#71786=(
GEOMETRIC_REPRESENTATION_CONTEXT(3)
GLOBAL_UNCERTAINTY_ASSIGNED_CONTEXT((#71774))
GLOBAL_UNIT_ASSIGNED_CONTEXT((#71796,#71798,#71799))
REPRESENTATION_CONTEXT('','3D')
);
#71795=(
GEOMETRIC_REPRESENTATION_CONTEXT(3)
GLOBAL_UNCERTAINTY_ASSIGNED_CONTEXT((#71783))
GLOBAL_UNIT_ASSIGNED_CONTEXT((#71796,#71798,#71799))
REPRESENTATION_CONTEXT('','3D')
);
#71796=(
LENGTH_UNIT()
NAMED_UNIT(*)
SI_UNIT(.MILLI.,.METRE.)
);
#71798=(
NAMED_UNIT(*)
PLANE_ANGLE_UNIT()
SI_UNIT($,.RADIAN.)
);
#71799=(
NAMED_UNIT(*)
SI_UNIT($,.STERADIAN.)
SOLID_ANGLE_UNIT()
);
#71802=SHAPE_DEFINITION_REPRESENTATION(#71813,#72018);
#71813=PRODUCT_DEFINITION_SHAPE('',$,#72030);
#72018=SHAPE_REPRESENTATION('',(#13854),#71786);
#72027=PRODUCT_DEFINITION_CONTEXT('part definition',#72062,'design');
#72030=PRODUCT_DEFINITION('Modular Carriage Plate 4.5 x 4.5',
'Modular Carriage Plate 4.5 x 4.5',#72041,#72027);
#72041=PRODUCT_DEFINITION_FORMATION('',$,#72066);
#72062=APPLICATION_CONTEXT(
'Core Data for Automotive Mechanical Design Process');
#72063=PRODUCT_CONTEXT('part definition',#72062,'mechanical');
#72066=PRODUCT('Modular Carriage Plate 4.5 x 4.5',
'Modular Carriage Plate 4.5 x 4.5',$,(#72063));
#72077=PRESENTATION_STYLE_ASSIGNMENT((#72088));
#72088=SURFACE_STYLE_USAGE(.BOTH.,#72099);
#72099=SURFACE_SIDE_STYLE('',(#72110));
#72110=SURFACE_STYLE_FILL_AREA(#72121);
#72121=FILL_AREA_STYLE('Opaque(222,225,230)',(#72132));
#72132=FILL_AREA_STYLE_COLOUR('Opaque(222,225,230)',#72143);
#72143=COLOUR_RGB('Opaque(222,225,230)', 0.66274510, 0.83137255, 0.94901961);
ENDSEC;
END-ISO-10303-21;
